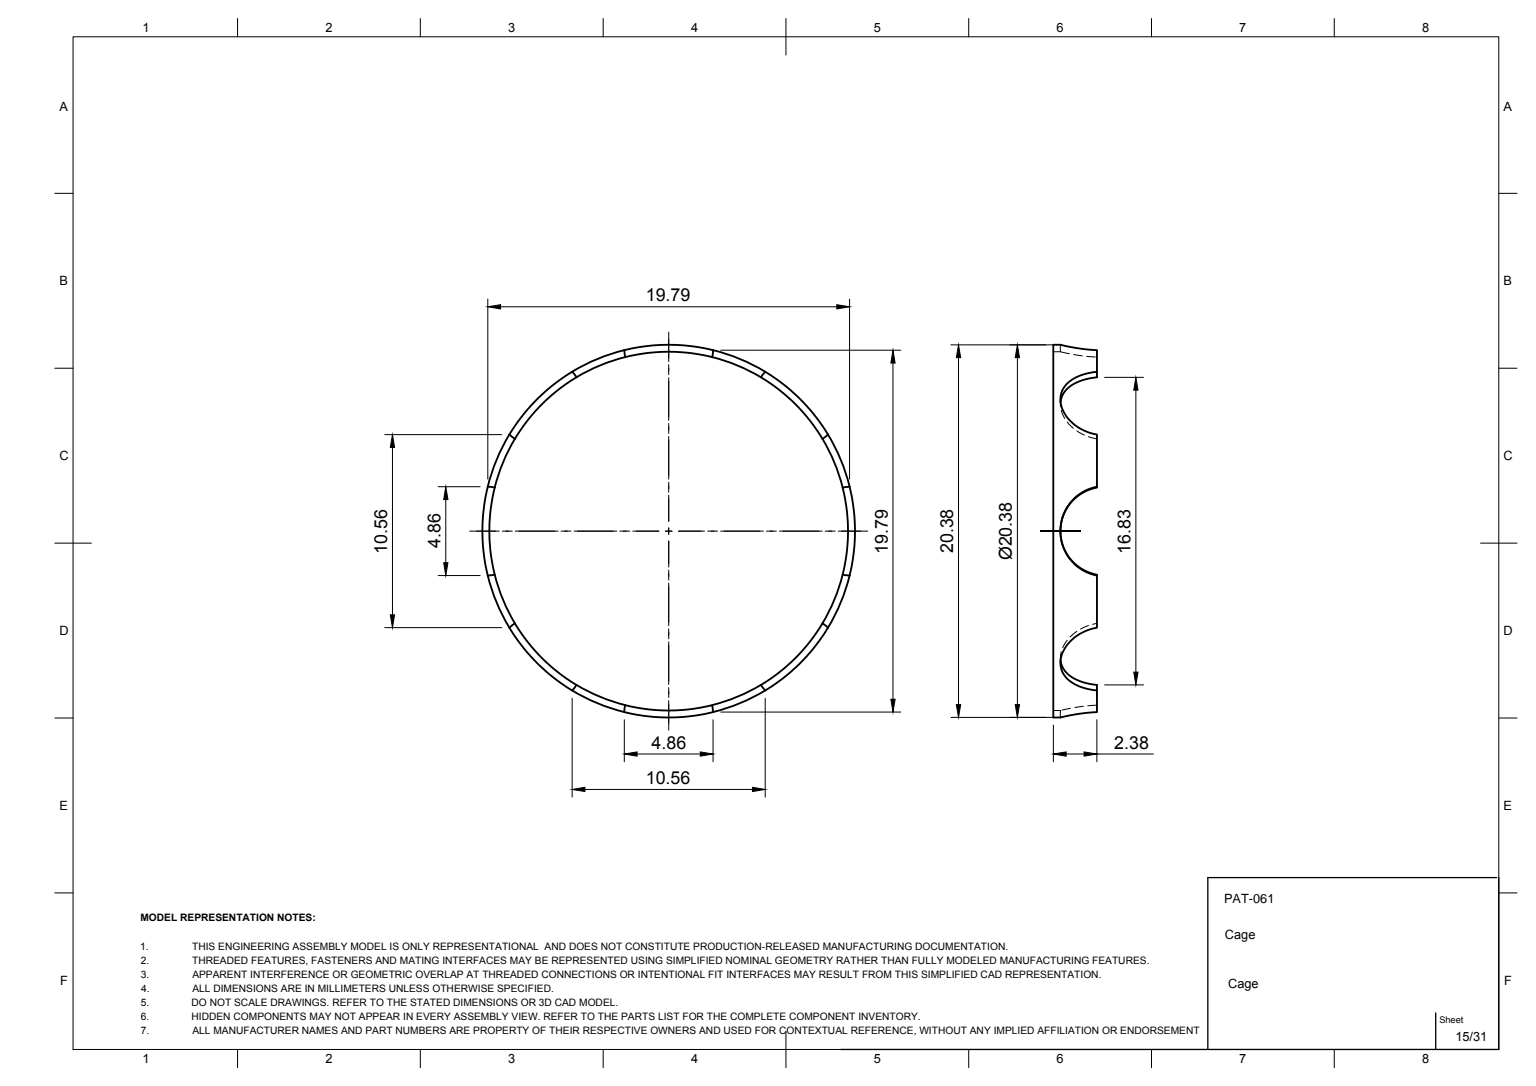
ISO-10303-21;
HEADER;
/* Generated by software containing ST-Developer
 * from STEP Tools, Inc. (www.steptools.com) 
 */

FILE_DESCRIPTION(
/* description */ ('Compact intermittent indexer'),
/* implementation_level */ '2;1');

FILE_NAME(
/* name */ 'Cage.step',
/* time_stamp */ '2026-10-29T16:32:17-07:00',
/* author */ (''),
/* organization */ (''),
/* preprocessor_version */ 'ST-DEVELOPER v20.2',
/* originating_system */ 'Autodesk Translation Framework v15.17.0.0',
/* authorisation */ '');

FILE_SCHEMA (('AUTOMOTIVE_DESIGN { 1 0 10303 214 3 1 1 }'));
ENDSEC;

DATA;
#10=MECHANICAL_DESIGN_GEOMETRIC_PRESENTATION_REPRESENTATION('',(#273),#10837);
#183=SPHERICAL_SURFACE('',#6247,0.247676);
#184=SPHERICAL_SURFACE('',#6263,0.247676);
#185=SPHERICAL_SURFACE('',#6268,0.247676);
#186=SPHERICAL_SURFACE('',#6273,0.247676);
#187=SPHERICAL_SURFACE('',#6278,0.247676);
#188=SPHERICAL_SURFACE('',#6283,0.247676);
#189=SPHERICAL_SURFACE('',#6288,0.247676);
#190=SPHERICAL_SURFACE('',#6296,0.247676);
#218=SHAPE_REPRESENTATION_RELATIONSHIP('SRR','None',#10953,#242);
#242=ADVANCED_BREP_SHAPE_REPRESENTATION('',(#304),#10820);
#273=STYLED_ITEM('',(#11166),#304);
#304=MANIFOLD_SOLID_BREP('Continuous crown cage',#5646);
#321=B_SPLINE_CURVE_WITH_KNOTS('',3,(#9240,#9241,#9242,#9243,#9244,#9245,
#9246,#9247,#9248,#9249,#9250,#9251,#9252,#9253,#9254,#9255,#9256,#9257,
#9258,#9259,#9260,#9261),.UNSPECIFIED.,.F.,.F.,(4,2,2,2,2,2,2,2,2,2,4),
(0.0473477652366656,0.126350602536658,0.189525903804987,0.252701205073317,
0.313298422430275,0.373895639787233,0.434492857144191,0.495090074501149,
0.558265375769478,0.621440677037807,0.7004435143378),.UNSPECIFIED.);
#322=B_SPLINE_CURVE_WITH_KNOTS('',3,(#9265,#9266,#9267,#9268,#9269,#9270,
#9271,#9272,#9273,#9274,#9275,#9276,#9277,#9278,#9279,#9280,#9281,#9282,
#9283,#9284,#9285,#9286),.UNSPECIFIED.,.F.,.F.,(4,2,2,2,2,2,2,2,2,2,4),
(0.0464897534940957,0.0852567806515119,0.170513561303024,0.246687263103517,
0.308657850341199,0.370628437578881,0.432599024816563,0.494569612054245,
0.570743313854739,0.656000094506251,0.694767121663666),.UNSPECIFIED.);
#323=B_SPLINE_CURVE_WITH_KNOTS('',3,(#9292,#9293,#9294,#9295,#9296,#9297,
#9298,#9299,#9300,#9301,#9302,#9303,#9304,#9305,#9306,#9307,#9308,#9309,
#9310,#9311,#9312,#9313),.UNSPECIFIED.,.F.,.F.,(4,2,2,2,2,2,2,2,2,2,4),
(0.0464897534940957,0.0852567806515118,0.170513561303024,0.246687263103517,
0.308657850341199,0.370628437578881,0.432599024816563,0.494569612054245,
0.570743313854738,0.65600009450625,0.694767121663666),.UNSPECIFIED.);
#324=B_SPLINE_CURVE_WITH_KNOTS('',3,(#9317,#9318,#9319,#9320,#9321,#9322,
#9323,#9324,#9325,#9326,#9327,#9328,#9329,#9330,#9331,#9332,#9333,#9334,
#9335,#9336,#9337,#9338),.UNSPECIFIED.,.F.,.F.,(4,2,2,2,2,2,2,2,2,2,4),
(0.0464897534940957,0.0852567806515119,0.170513561303024,0.246687263103517,
0.308657850341199,0.370628437578881,0.432599024816563,0.494569612054245,
0.570743313854739,0.656000094506251,0.694767121663666),.UNSPECIFIED.);
#325=B_SPLINE_CURVE_WITH_KNOTS('',3,(#9342,#9343,#9344,#9345,#9346,#9347,
#9348,#9349,#9350,#9351,#9352,#9353),.UNSPECIFIED.,.F.,.F.,(4,2,2,2,2,4),
(0.0464897534940957,0.0852567806515119,0.170513561303024,0.246687263103517,
0.308657850341199,0.370628437578881),.UNSPECIFIED.);
#326=B_SPLINE_CURVE_WITH_KNOTS('',3,(#9358,#9359,#9360,#9361,#9362,#9363,
#9364,#9365,#9366,#9367,#9368,#9369),.UNSPECIFIED.,.F.,.F.,(4,2,2,2,2,4),
(0.370628437578881,0.432599024816563,0.494569612054245,0.570743313854738,
0.65600009450625,0.694767121663666),.UNSPECIFIED.);
#327=B_SPLINE_CURVE_WITH_KNOTS('',3,(#9373,#9374,#9375,#9376,#9377,#9378,
#9379,#9380,#9381,#9382,#9383,#9384,#9385,#9386,#9387,#9388,#9389,#9390,
#9391,#9392,#9393,#9394),.UNSPECIFIED.,.F.,.F.,(4,2,2,2,2,2,2,2,2,2,4),
(0.0464897534940957,0.0852567806515121,0.170513561303024,0.246687263103518,
0.308657850341199,0.370628437578881,0.432599024816563,0.494569612054245,
0.570743313854738,0.65600009450625,0.694767121663666),.UNSPECIFIED.);
#328=B_SPLINE_CURVE_WITH_KNOTS('',3,(#9398,#9399,#9400,#9401,#9402,#9403,
#9404,#9405,#9406,#9407,#9408,#9409,#9410,#9411,#9412,#9413,#9414,#9415,
#9416,#9417,#9418,#9419),.UNSPECIFIED.,.F.,.F.,(4,2,2,2,2,2,2,2,2,2,4),
(0.0464897534940957,0.0852567806515119,0.170513561303024,0.246687263103517,
0.308657850341199,0.370628437578881,0.432599024816563,0.494569612054245,
0.570743313854738,0.65600009450625,0.694767121663667),.UNSPECIFIED.);
#329=B_SPLINE_CURVE_WITH_KNOTS('',3,(#9423,#9424,#9425,#9426,#9427,#9428,
#9429,#9430,#9431,#9432,#9433,#9434,#9435,#9436,#9437,#9438,#9439,#9440,
#9441,#9442,#9443,#9444),.UNSPECIFIED.,.F.,.F.,(4,2,2,2,2,2,2,2,2,2,4),
(0.0464897534940957,0.0852567806515119,0.170513561303024,0.246687263103517,
0.308657850341199,0.370628437578881,0.432599024816563,0.494569612054245,
0.570743313854738,0.65600009450625,0.694767121663666),.UNSPECIFIED.);
#330=B_SPLINE_CURVE_WITH_KNOTS('',3,(#9448,#9449,#9450,#9451,#9452,#9453,
#9454,#9455,#9456,#9457,#9458,#9459,#9460,#9461,#9462,#9463,#9464,#9465,
#9466,#9467,#9468,#9469),.UNSPECIFIED.,.F.,.F.,(4,2,2,2,2,2,2,2,2,2,4),
(0.0464897534940957,0.0852567806515119,0.170513561303024,0.246687263103517,
0.308657850341199,0.370628437578881,0.432599024816563,0.494569612054245,
0.570743313854739,0.656000094506251,0.694767121663667),.UNSPECIFIED.);
#331=B_SPLINE_CURVE_WITH_KNOTS('',3,(#9477,#9478,#9479,#9480,#9481,#9482,
#9483,#9484,#9485,#9486,#9487,#9488,#9489,#9490,#9491,#9492,#9493,#9494,
#9495,#9496,#9497,#9498),.UNSPECIFIED.,.F.,.F.,(4,2,2,2,2,2,2,2,2,2,4),
(0.0473477652366656,0.126350602536658,0.189525903804987,0.252701205073316,
0.313298422430274,0.373895639787232,0.434492857144191,0.495090074501149,
0.558265375769478,0.621440677037807,0.7004435143378),.UNSPECIFIED.);
#332=B_SPLINE_CURVE_WITH_KNOTS('',3,(#9506,#9507,#9508,#9509,#9510,#9511,
#9512,#9513,#9514,#9515,#9516,#9517,#9518,#9519,#9520,#9521,#9522,#9523,
#9524,#9525,#9526,#9527),.UNSPECIFIED.,.F.,.F.,(4,2,2,2,2,2,2,2,2,2,4),
(0.0473477652366656,0.126350602536658,0.189525903804987,0.252701205073317,
0.313298422430275,0.373895639787233,0.434492857144191,0.495090074501149,
0.558265375769478,0.621440677037807,0.7004435143378),.UNSPECIFIED.);
#333=B_SPLINE_CURVE_WITH_KNOTS('',3,(#9536,#9537,#9538,#9539,#9540,#9541,
#9542,#9543,#9544,#9545,#9546,#9547),.UNSPECIFIED.,.F.,.F.,(4,2,2,2,2,4),
(0.0473477652366656,0.126350602536658,0.189525903804987,0.252701205073316,
0.313298422430275,0.373895639787233),.UNSPECIFIED.);
#334=B_SPLINE_CURVE_WITH_KNOTS('',3,(#9549,#9550,#9551,#9552,#9553,#9554,
#9555,#9556,#9557,#9558,#9559,#9560),.UNSPECIFIED.,.F.,.F.,(4,2,2,2,2,4),
(0.373895639787233,0.434492857144191,0.495090074501149,0.558265375769478,
0.621440677037807,0.7004435143378),.UNSPECIFIED.);
#335=B_SPLINE_CURVE_WITH_KNOTS('',3,(#9567,#9568,#9569,#9570,#9571,#9572,
#9573,#9574,#9575,#9576,#9577,#9578,#9579,#9580,#9581,#9582,#9583,#9584,
#9585,#9586,#9587,#9588),.UNSPECIFIED.,.F.,.F.,(4,2,2,2,2,2,2,2,2,2,4),
(0.0473477652366656,0.126350602536658,0.189525903804987,0.252701205073316,
0.313298422430275,0.373895639787233,0.434492857144191,0.495090074501149,
0.558265375769478,0.621440677037807,0.7004435143378),.UNSPECIFIED.);
#336=B_SPLINE_CURVE_WITH_KNOTS('',3,(#9596,#9597,#9598,#9599,#9600,#9601,
#9602,#9603,#9604,#9605,#9606,#9607,#9608,#9609,#9610,#9611,#9612,#9613,
#9614,#9615,#9616,#9617),.UNSPECIFIED.,.F.,.F.,(4,2,2,2,2,2,2,2,2,2,4),
(0.0473477652366656,0.126350602536658,0.189525903804987,0.252701205073317,
0.313298422430275,0.373895639787233,0.434492857144191,0.495090074501149,
0.558265375769478,0.621440677037807,0.7004435143378),.UNSPECIFIED.);
#337=B_SPLINE_CURVE_WITH_KNOTS('',3,(#9625,#9626,#9627,#9628,#9629,#9630,
#9631,#9632,#9633,#9634,#9635,#9636,#9637,#9638,#9639,#9640,#9641,#9642,
#9643,#9644,#9645,#9646),.UNSPECIFIED.,.F.,.F.,(4,2,2,2,2,2,2,2,2,2,4),
(0.0473477652366656,0.126350602536658,0.189525903804987,0.252701205073316,
0.313298422430275,0.373895639787233,0.434492857144191,0.495090074501149,
0.558265375769478,0.621440677037807,0.7004435143378),.UNSPECIFIED.);
#338=B_SPLINE_CURVE_WITH_KNOTS('',3,(#9655,#9656,#9657,#9658,#9659,#9660,
#9661,#9662,#9663,#9664,#9665,#9666,#9667,#9668,#9669,#9670,#9671,#9672,
#9673,#9674,#9675,#9676),.UNSPECIFIED.,.F.,.F.,(4,2,2,2,2,2,2,2,2,2,4),
(0.0473477652366656,0.126350602536658,0.189525903804987,0.252701205073317,
0.313298422430275,0.373895639787233,0.434492857144191,0.495090074501149,
0.558265375769478,0.621440677037807,0.7004435143378),.UNSPECIFIED.);
#427=FACE_BOUND('',#1222,.T.);
#543=PLANE('',#6260);
#544=PLANE('',#6265);
#545=PLANE('',#6270);
#546=PLANE('',#6275);
#547=PLANE('',#6280);
#548=PLANE('',#6285);
#549=PLANE('',#6294);
#550=PLANE('',#6298);
#551=PLANE('',#6299);
#802=FACE_OUTER_BOUND('',#1204,.T.);
#803=FACE_OUTER_BOUND('',#1205,.T.);
#804=FACE_OUTER_BOUND('',#1206,.T.);
#805=FACE_OUTER_BOUND('',#1207,.T.);
#806=FACE_OUTER_BOUND('',#1208,.T.);
#807=FACE_OUTER_BOUND('',#1209,.T.);
#808=FACE_OUTER_BOUND('',#1210,.T.);
#809=FACE_OUTER_BOUND('',#1211,.T.);
#810=FACE_OUTER_BOUND('',#1212,.T.);
#811=FACE_OUTER_BOUND('',#1213,.T.);
#812=FACE_OUTER_BOUND('',#1214,.T.);
#813=FACE_OUTER_BOUND('',#1215,.T.);
#814=FACE_OUTER_BOUND('',#1216,.T.);
#815=FACE_OUTER_BOUND('',#1217,.T.);
#816=FACE_OUTER_BOUND('',#1218,.T.);
#817=FACE_OUTER_BOUND('',#1219,.T.);
#818=FACE_OUTER_BOUND('',#1220,.T.);
#819=FACE_OUTER_BOUND('',#1221,.T.);
#820=FACE_OUTER_BOUND('',#1223,.T.);
#1204=EDGE_LOOP('',(#4308,#4309,#4310,#4311));
#1205=EDGE_LOOP('',(#4312,#4313,#4314,#4315,#4316,#4317,#4318,#4319,#4320,
#4321,#4322,#4323,#4324,#4325,#4326,#4327,#4328,#4329,#4330,#4331));
#1206=EDGE_LOOP('',(#4332,#4333,#4334,#4335));
#1207=EDGE_LOOP('',(#4336,#4337,#4338,#4339));
#1208=EDGE_LOOP('',(#4340,#4341,#4342,#4343));
#1209=EDGE_LOOP('',(#4344,#4345,#4346,#4347));
#1210=EDGE_LOOP('',(#4348,#4349,#4350,#4351));
#1211=EDGE_LOOP('',(#4352,#4353,#4354,#4355,#4356,#4357));
#1212=EDGE_LOOP('',(#4358,#4359,#4360,#4361));
#1213=EDGE_LOOP('',(#4362,#4363,#4364,#4365));
#1214=EDGE_LOOP('',(#4366,#4367,#4368,#4369));
#1215=EDGE_LOOP('',(#4370,#4371,#4372,#4373));
#1216=EDGE_LOOP('',(#4374,#4375,#4376,#4377));
#1217=EDGE_LOOP('',(#4378,#4379,#4380,#4381));
#1218=EDGE_LOOP('',(#4382,#4383,#4384,#4385,#4386,#4387,#4388,#4389,#4390,
#4391,#4392,#4393,#4394,#4395,#4396,#4397,#4398,#4399,#4400,#4401));
#1219=EDGE_LOOP('',(#4402,#4403,#4404,#4405));
#1220=EDGE_LOOP('',(#4406,#4407,#4408,#4409));
#1221=EDGE_LOOP('',(#4410));
#1222=EDGE_LOOP('',(#4411));
#1223=EDGE_LOOP('',(#4412,#4413,#4414,#4415));
#1574=LINE('',#9355,#1932);
#1575=LINE('',#9651,#1933);
#1932=VECTOR('',#7460,1.019052);
#1933=VECTOR('',#7537,0.980948);
#2304=CIRCLE('',#6248,0.243053047864041);
#2305=CIRCLE('',#6249,0.243053047864041);
#2306=CIRCLE('',#6251,1.019052);
#2307=CIRCLE('',#6252,1.019052);
#2308=CIRCLE('',#6253,1.019052);
#2309=CIRCLE('',#6254,1.019052);
#2310=CIRCLE('',#6255,1.019052);
#2311=CIRCLE('',#6256,1.019052);
#2312=CIRCLE('',#6257,1.019052);
#2313=CIRCLE('',#6258,1.019052);
#2314=CIRCLE('',#6259,1.019052);
#2315=CIRCLE('',#6261,0.980948);
#2316=CIRCLE('',#6262,0.243053047864041);
#2317=CIRCLE('',#6264,0.243053047864041);
#2318=CIRCLE('',#6266,0.980948);
#2319=CIRCLE('',#6267,0.243053047864041);
#2320=CIRCLE('',#6269,0.243053047864041);
#2321=CIRCLE('',#6271,0.980948);
#2322=CIRCLE('',#6272,0.243053047864041);
#2323=CIRCLE('',#6274,0.243053047864041);
#2324=CIRCLE('',#6276,0.980948);
#2325=CIRCLE('',#6277,0.243053047864041);
#2326=CIRCLE('',#6279,0.243053047864041);
#2327=CIRCLE('',#6281,0.980948);
#2328=CIRCLE('',#6282,0.243053047864041);
#2329=CIRCLE('',#6284,0.243053047864041);
#2330=CIRCLE('',#6286,0.980948);
#2331=CIRCLE('',#6287,0.243053047864041);
#2332=CIRCLE('',#6289,0.243053047864041);
#2333=CIRCLE('',#6291,0.980948);
#2334=CIRCLE('',#6292,0.980948);
#2335=CIRCLE('',#6293,0.980948);
#2336=CIRCLE('',#6295,0.243053047864041);
#2337=CIRCLE('',#6297,0.243053047864041);
#2690=VERTEX_POINT('',#9238);
#2691=VERTEX_POINT('',#9239);
#2692=VERTEX_POINT('',#9262);
#2693=VERTEX_POINT('',#9264);
#2694=VERTEX_POINT('',#9289);
#2695=VERTEX_POINT('',#9291);
#2696=VERTEX_POINT('',#9314);
#2697=VERTEX_POINT('',#9316);
#2698=VERTEX_POINT('',#9339);
#2699=VERTEX_POINT('',#9341);
#2700=VERTEX_POINT('',#9354);
#2701=VERTEX_POINT('',#9357);
#2702=VERTEX_POINT('',#9370);
#2703=VERTEX_POINT('',#9372);
#2704=VERTEX_POINT('',#9395);
#2705=VERTEX_POINT('',#9397);
#2706=VERTEX_POINT('',#9420);
#2707=VERTEX_POINT('',#9422);
#2708=VERTEX_POINT('',#9445);
#2709=VERTEX_POINT('',#9447);
#2710=VERTEX_POINT('',#9472);
#2711=VERTEX_POINT('',#9476);
#2712=VERTEX_POINT('',#9501);
#2713=VERTEX_POINT('',#9505);
#2714=VERTEX_POINT('',#9530);
#2715=VERTEX_POINT('',#9534);
#2716=VERTEX_POINT('',#9535);
#2717=VERTEX_POINT('',#9562);
#2718=VERTEX_POINT('',#9566);
#2719=VERTEX_POINT('',#9591);
#2720=VERTEX_POINT('',#9595);
#2721=VERTEX_POINT('',#9620);
#2722=VERTEX_POINT('',#9624);
#2723=VERTEX_POINT('',#9649);
#2724=VERTEX_POINT('',#9652);
#2725=VERTEX_POINT('',#9654);
#3276=EDGE_CURVE('',#2690,#2691,#321,.T.);
#3277=EDGE_CURVE('',#2692,#2690,#2304,.T.);
#3278=EDGE_CURVE('',#2693,#2692,#322,.T.);
#3279=EDGE_CURVE('',#2691,#2693,#2305,.T.);
#3280=EDGE_CURVE('',#2694,#2692,#2306,.T.);
#3281=EDGE_CURVE('',#2694,#2695,#323,.T.);
#3282=EDGE_CURVE('',#2696,#2695,#2307,.T.);
#3283=EDGE_CURVE('',#2696,#2697,#324,.T.);
#3284=EDGE_CURVE('',#2698,#2697,#2308,.T.);
#3285=EDGE_CURVE('',#2698,#2699,#325,.T.);
#3286=EDGE_CURVE('',#2699,#2700,#1574,.T.);
#3287=EDGE_CURVE('',#2700,#2700,#2309,.T.);
#3288=EDGE_CURVE('',#2699,#2701,#326,.T.);
#3289=EDGE_CURVE('',#2702,#2701,#2310,.T.);
#3290=EDGE_CURVE('',#2702,#2703,#327,.T.);
#3291=EDGE_CURVE('',#2704,#2703,#2311,.T.);
#3292=EDGE_CURVE('',#2704,#2705,#328,.T.);
#3293=EDGE_CURVE('',#2706,#2705,#2312,.T.);
#3294=EDGE_CURVE('',#2706,#2707,#329,.T.);
#3295=EDGE_CURVE('',#2708,#2707,#2313,.T.);
#3296=EDGE_CURVE('',#2708,#2709,#330,.T.);
#3297=EDGE_CURVE('',#2693,#2709,#2314,.T.);
#3298=EDGE_CURVE('',#2690,#2710,#2315,.T.);
#3299=EDGE_CURVE('',#2710,#2694,#2316,.T.);
#3300=EDGE_CURVE('',#2711,#2710,#331,.T.);
#3301=EDGE_CURVE('',#2695,#2711,#2317,.T.);
#3302=EDGE_CURVE('',#2711,#2712,#2318,.T.);
#3303=EDGE_CURVE('',#2712,#2696,#2319,.T.);
#3304=EDGE_CURVE('',#2713,#2712,#332,.T.);
#3305=EDGE_CURVE('',#2697,#2713,#2320,.T.);
#3306=EDGE_CURVE('',#2713,#2714,#2321,.T.);
#3307=EDGE_CURVE('',#2714,#2698,#2322,.T.);
#3308=EDGE_CURVE('',#2715,#2716,#333,.T.);
#3309=EDGE_CURVE('',#2701,#2715,#2323,.T.);
#3310=EDGE_CURVE('',#2716,#2714,#334,.T.);
#3311=EDGE_CURVE('',#2715,#2717,#2324,.T.);
#3312=EDGE_CURVE('',#2717,#2702,#2325,.T.);
#3313=EDGE_CURVE('',#2718,#2717,#335,.T.);
#3314=EDGE_CURVE('',#2703,#2718,#2326,.T.);
#3315=EDGE_CURVE('',#2718,#2719,#2327,.T.);
#3316=EDGE_CURVE('',#2719,#2704,#2328,.T.);
#3317=EDGE_CURVE('',#2720,#2719,#336,.T.);
#3318=EDGE_CURVE('',#2705,#2720,#2329,.T.);
#3319=EDGE_CURVE('',#2720,#2721,#2330,.T.);
#3320=EDGE_CURVE('',#2721,#2706,#2331,.T.);
#3321=EDGE_CURVE('',#2722,#2721,#337,.T.);
#3322=EDGE_CURVE('',#2707,#2722,#2332,.T.);
#3323=EDGE_CURVE('',#2723,#2723,#2333,.T.);
#3324=EDGE_CURVE('',#2723,#2716,#1575,.T.);
#3325=EDGE_CURVE('',#2724,#2691,#2334,.T.);
#3326=EDGE_CURVE('',#2724,#2725,#338,.T.);
#3327=EDGE_CURVE('',#2722,#2725,#2335,.T.);
#3328=EDGE_CURVE('',#2709,#2724,#2336,.T.);
#3329=EDGE_CURVE('',#2725,#2708,#2337,.T.);
#4308=ORIENTED_EDGE('',*,*,#3276,.F.);
#4309=ORIENTED_EDGE('',*,*,#3277,.F.);
#4310=ORIENTED_EDGE('',*,*,#3278,.F.);
#4311=ORIENTED_EDGE('',*,*,#3279,.F.);
#4312=ORIENTED_EDGE('',*,*,#3278,.T.);
#4313=ORIENTED_EDGE('',*,*,#3280,.F.);
#4314=ORIENTED_EDGE('',*,*,#3281,.T.);
#4315=ORIENTED_EDGE('',*,*,#3282,.F.);
#4316=ORIENTED_EDGE('',*,*,#3283,.T.);
#4317=ORIENTED_EDGE('',*,*,#3284,.F.);
#4318=ORIENTED_EDGE('',*,*,#3285,.T.);
#4319=ORIENTED_EDGE('',*,*,#3286,.T.);
#4320=ORIENTED_EDGE('',*,*,#3287,.F.);
#4321=ORIENTED_EDGE('',*,*,#3286,.F.);
#4322=ORIENTED_EDGE('',*,*,#3288,.T.);
#4323=ORIENTED_EDGE('',*,*,#3289,.F.);
#4324=ORIENTED_EDGE('',*,*,#3290,.T.);
#4325=ORIENTED_EDGE('',*,*,#3291,.F.);
#4326=ORIENTED_EDGE('',*,*,#3292,.T.);
#4327=ORIENTED_EDGE('',*,*,#3293,.F.);
#4328=ORIENTED_EDGE('',*,*,#3294,.T.);
#4329=ORIENTED_EDGE('',*,*,#3295,.F.);
#4330=ORIENTED_EDGE('',*,*,#3296,.T.);
#4331=ORIENTED_EDGE('',*,*,#3297,.F.);
#4332=ORIENTED_EDGE('',*,*,#3277,.T.);
#4333=ORIENTED_EDGE('',*,*,#3298,.T.);
#4334=ORIENTED_EDGE('',*,*,#3299,.T.);
#4335=ORIENTED_EDGE('',*,*,#3280,.T.);
#4336=ORIENTED_EDGE('',*,*,#3300,.F.);
#4337=ORIENTED_EDGE('',*,*,#3301,.F.);
#4338=ORIENTED_EDGE('',*,*,#3281,.F.);
#4339=ORIENTED_EDGE('',*,*,#3299,.F.);
#4340=ORIENTED_EDGE('',*,*,#3301,.T.);
#4341=ORIENTED_EDGE('',*,*,#3302,.T.);
#4342=ORIENTED_EDGE('',*,*,#3303,.T.);
#4343=ORIENTED_EDGE('',*,*,#3282,.T.);
#4344=ORIENTED_EDGE('',*,*,#3304,.F.);
#4345=ORIENTED_EDGE('',*,*,#3305,.F.);
#4346=ORIENTED_EDGE('',*,*,#3283,.F.);
#4347=ORIENTED_EDGE('',*,*,#3303,.F.);
#4348=ORIENTED_EDGE('',*,*,#3305,.T.);
#4349=ORIENTED_EDGE('',*,*,#3306,.T.);
#4350=ORIENTED_EDGE('',*,*,#3307,.T.);
#4351=ORIENTED_EDGE('',*,*,#3284,.T.);
#4352=ORIENTED_EDGE('',*,*,#3308,.F.);
#4353=ORIENTED_EDGE('',*,*,#3309,.F.);
#4354=ORIENTED_EDGE('',*,*,#3288,.F.);
#4355=ORIENTED_EDGE('',*,*,#3285,.F.);
#4356=ORIENTED_EDGE('',*,*,#3307,.F.);
#4357=ORIENTED_EDGE('',*,*,#3310,.F.);
#4358=ORIENTED_EDGE('',*,*,#3309,.T.);
#4359=ORIENTED_EDGE('',*,*,#3311,.T.);
#4360=ORIENTED_EDGE('',*,*,#3312,.T.);
#4361=ORIENTED_EDGE('',*,*,#3289,.T.);
#4362=ORIENTED_EDGE('',*,*,#3313,.F.);
#4363=ORIENTED_EDGE('',*,*,#3314,.F.);
#4364=ORIENTED_EDGE('',*,*,#3290,.F.);
#4365=ORIENTED_EDGE('',*,*,#3312,.F.);
#4366=ORIENTED_EDGE('',*,*,#3314,.T.);
#4367=ORIENTED_EDGE('',*,*,#3315,.T.);
#4368=ORIENTED_EDGE('',*,*,#3316,.T.);
#4369=ORIENTED_EDGE('',*,*,#3291,.T.);
#4370=ORIENTED_EDGE('',*,*,#3317,.F.);
#4371=ORIENTED_EDGE('',*,*,#3318,.F.);
#4372=ORIENTED_EDGE('',*,*,#3292,.F.);
#4373=ORIENTED_EDGE('',*,*,#3316,.F.);
#4374=ORIENTED_EDGE('',*,*,#3318,.T.);
#4375=ORIENTED_EDGE('',*,*,#3319,.T.);
#4376=ORIENTED_EDGE('',*,*,#3320,.T.);
#4377=ORIENTED_EDGE('',*,*,#3293,.T.);
#4378=ORIENTED_EDGE('',*,*,#3294,.F.);
#4379=ORIENTED_EDGE('',*,*,#3320,.F.);
#4380=ORIENTED_EDGE('',*,*,#3321,.F.);
#4381=ORIENTED_EDGE('',*,*,#3322,.F.);
#4382=ORIENTED_EDGE('',*,*,#3323,.F.);
#4383=ORIENTED_EDGE('',*,*,#3324,.T.);
#4384=ORIENTED_EDGE('',*,*,#3310,.T.);
#4385=ORIENTED_EDGE('',*,*,#3306,.F.);
#4386=ORIENTED_EDGE('',*,*,#3304,.T.);
#4387=ORIENTED_EDGE('',*,*,#3302,.F.);
#4388=ORIENTED_EDGE('',*,*,#3300,.T.);
#4389=ORIENTED_EDGE('',*,*,#3298,.F.);
#4390=ORIENTED_EDGE('',*,*,#3276,.T.);
#4391=ORIENTED_EDGE('',*,*,#3325,.F.);
#4392=ORIENTED_EDGE('',*,*,#3326,.T.);
#4393=ORIENTED_EDGE('',*,*,#3327,.F.);
#4394=ORIENTED_EDGE('',*,*,#3321,.T.);
#4395=ORIENTED_EDGE('',*,*,#3319,.F.);
#4396=ORIENTED_EDGE('',*,*,#3317,.T.);
#4397=ORIENTED_EDGE('',*,*,#3315,.F.);
#4398=ORIENTED_EDGE('',*,*,#3313,.T.);
#4399=ORIENTED_EDGE('',*,*,#3311,.F.);
#4400=ORIENTED_EDGE('',*,*,#3308,.T.);
#4401=ORIENTED_EDGE('',*,*,#3324,.F.);
#4402=ORIENTED_EDGE('',*,*,#3279,.T.);
#4403=ORIENTED_EDGE('',*,*,#3297,.T.);
#4404=ORIENTED_EDGE('',*,*,#3328,.T.);
#4405=ORIENTED_EDGE('',*,*,#3325,.T.);
#4406=ORIENTED_EDGE('',*,*,#3296,.F.);
#4407=ORIENTED_EDGE('',*,*,#3329,.F.);
#4408=ORIENTED_EDGE('',*,*,#3326,.F.);
#4409=ORIENTED_EDGE('',*,*,#3328,.F.);
#4410=ORIENTED_EDGE('',*,*,#3287,.T.);
#4411=ORIENTED_EDGE('',*,*,#3323,.T.);
#4412=ORIENTED_EDGE('',*,*,#3322,.T.);
#4413=ORIENTED_EDGE('',*,*,#3327,.T.);
#4414=ORIENTED_EDGE('',*,*,#3329,.T.);
#4415=ORIENTED_EDGE('',*,*,#3295,.T.);
#5232=CYLINDRICAL_SURFACE('',#6250,1.019052);
#5233=CYLINDRICAL_SURFACE('',#6290,0.980948);
#5445=ADVANCED_FACE('',(#802),#183,.F.);
#5446=ADVANCED_FACE('',(#803),#5232,.T.);
#5447=ADVANCED_FACE('',(#804),#543,.T.);
#5448=ADVANCED_FACE('',(#805),#184,.F.);
#5449=ADVANCED_FACE('',(#806),#544,.T.);
#5450=ADVANCED_FACE('',(#807),#185,.F.);
#5451=ADVANCED_FACE('',(#808),#545,.T.);
#5452=ADVANCED_FACE('',(#809),#186,.F.);
#5453=ADVANCED_FACE('',(#810),#546,.T.);
#5454=ADVANCED_FACE('',(#811),#187,.F.);
#5455=ADVANCED_FACE('',(#812),#547,.T.);
#5456=ADVANCED_FACE('',(#813),#188,.F.);
#5457=ADVANCED_FACE('',(#814),#548,.T.);
#5458=ADVANCED_FACE('',(#815),#189,.F.);
#5459=ADVANCED_FACE('',(#816),#5233,.F.);
#5460=ADVANCED_FACE('',(#817),#549,.T.);
#5461=ADVANCED_FACE('',(#818),#190,.F.);
#5462=ADVANCED_FACE('',(#819,#427),#550,.T.);
#5463=ADVANCED_FACE('',(#820),#551,.T.);
#5646=CLOSED_SHELL('',(#5445,#5446,#5447,#5448,#5449,#5450,#5451,#5452,
#5453,#5454,#5455,#5456,#5457,#5458,#5459,#5460,#5461,#5462,#5463));
#6246=AXIS2_PLACEMENT_3D('',#9236,#7444,#7445);
#6247=AXIS2_PLACEMENT_3D('',#9237,#7446,#7447);
#6248=AXIS2_PLACEMENT_3D('',#9263,#7448,#7449);
#6249=AXIS2_PLACEMENT_3D('',#9287,#7450,#7451);
#6250=AXIS2_PLACEMENT_3D('',#9288,#7452,#7453);
#6251=AXIS2_PLACEMENT_3D('',#9290,#7454,#7455);
#6252=AXIS2_PLACEMENT_3D('',#9315,#7456,#7457);
#6253=AXIS2_PLACEMENT_3D('',#9340,#7458,#7459);
#6254=AXIS2_PLACEMENT_3D('',#9356,#7461,#7462);
#6255=AXIS2_PLACEMENT_3D('',#9371,#7463,#7464);
#6256=AXIS2_PLACEMENT_3D('',#9396,#7465,#7466);
#6257=AXIS2_PLACEMENT_3D('',#9421,#7467,#7468);
#6258=AXIS2_PLACEMENT_3D('',#9446,#7469,#7470);
#6259=AXIS2_PLACEMENT_3D('',#9470,#7471,#7472);
#6260=AXIS2_PLACEMENT_3D('',#9471,#7473,#7474);
#6261=AXIS2_PLACEMENT_3D('',#9473,#7475,#7476);
#6262=AXIS2_PLACEMENT_3D('',#9474,#7477,#7478);
#6263=AXIS2_PLACEMENT_3D('',#9475,#7479,#7480);
#6264=AXIS2_PLACEMENT_3D('',#9499,#7481,#7482);
#6265=AXIS2_PLACEMENT_3D('',#9500,#7483,#7484);
#6266=AXIS2_PLACEMENT_3D('',#9502,#7485,#7486);
#6267=AXIS2_PLACEMENT_3D('',#9503,#7487,#7488);
#6268=AXIS2_PLACEMENT_3D('',#9504,#7489,#7490);
#6269=AXIS2_PLACEMENT_3D('',#9528,#7491,#7492);
#6270=AXIS2_PLACEMENT_3D('',#9529,#7493,#7494);
#6271=AXIS2_PLACEMENT_3D('',#9531,#7495,#7496);
#6272=AXIS2_PLACEMENT_3D('',#9532,#7497,#7498);
#6273=AXIS2_PLACEMENT_3D('',#9533,#7499,#7500);
#6274=AXIS2_PLACEMENT_3D('',#9548,#7501,#7502);
#6275=AXIS2_PLACEMENT_3D('',#9561,#7503,#7504);
#6276=AXIS2_PLACEMENT_3D('',#9563,#7505,#7506);
#6277=AXIS2_PLACEMENT_3D('',#9564,#7507,#7508);
#6278=AXIS2_PLACEMENT_3D('',#9565,#7509,#7510);
#6279=AXIS2_PLACEMENT_3D('',#9589,#7511,#7512);
#6280=AXIS2_PLACEMENT_3D('',#9590,#7513,#7514);
#6281=AXIS2_PLACEMENT_3D('',#9592,#7515,#7516);
#6282=AXIS2_PLACEMENT_3D('',#9593,#7517,#7518);
#6283=AXIS2_PLACEMENT_3D('',#9594,#7519,#7520);
#6284=AXIS2_PLACEMENT_3D('',#9618,#7521,#7522);
#6285=AXIS2_PLACEMENT_3D('',#9619,#7523,#7524);
#6286=AXIS2_PLACEMENT_3D('',#9621,#7525,#7526);
#6287=AXIS2_PLACEMENT_3D('',#9622,#7527,#7528);
#6288=AXIS2_PLACEMENT_3D('',#9623,#7529,#7530);
#6289=AXIS2_PLACEMENT_3D('',#9647,#7531,#7532);
#6290=AXIS2_PLACEMENT_3D('',#9648,#7533,#7534);
#6291=AXIS2_PLACEMENT_3D('',#9650,#7535,#7536);
#6292=AXIS2_PLACEMENT_3D('',#9653,#7538,#7539);
#6293=AXIS2_PLACEMENT_3D('',#9677,#7540,#7541);
#6294=AXIS2_PLACEMENT_3D('',#9678,#7542,#7543);
#6295=AXIS2_PLACEMENT_3D('',#9679,#7544,#7545);
#6296=AXIS2_PLACEMENT_3D('',#9680,#7546,#7547);
#6297=AXIS2_PLACEMENT_3D('',#9681,#7548,#7549);
#6298=AXIS2_PLACEMENT_3D('',#9682,#7550,#7551);
#6299=AXIS2_PLACEMENT_3D('',#9683,#7552,#7553);
#7444=DIRECTION('axis',(0.,0.,1.));
#7445=DIRECTION('refdir',(1.,0.,0.));
#7446=DIRECTION('center_axis',(0.,0.,1.));
#7447=DIRECTION('ref_axis',(1.,0.,0.));
#7448=DIRECTION('center_axis',(0.,-1.,0.));
#7449=DIRECTION('ref_axis',(0.,0.,-1.));
#7450=DIRECTION('center_axis',(0.,-1.,0.));
#7451=DIRECTION('ref_axis',(0.,0.,-1.));
#7452=DIRECTION('center_axis',(0.,1.,0.));
#7453=DIRECTION('ref_axis',(1.,0.,0.));
#7454=DIRECTION('center_axis',(0.,1.,0.));
#7455=DIRECTION('ref_axis',(1.,0.,0.));
#7456=DIRECTION('center_axis',(0.,1.,0.));
#7457=DIRECTION('ref_axis',(1.,0.,0.));
#7458=DIRECTION('center_axis',(0.,1.,0.));
#7459=DIRECTION('ref_axis',(1.,0.,0.));
#7460=DIRECTION('',(0.,-1.,0.));
#7461=DIRECTION('center_axis',(0.,-1.,0.));
#7462=DIRECTION('ref_axis',(1.,0.,0.));
#7463=DIRECTION('center_axis',(0.,1.,0.));
#7464=DIRECTION('ref_axis',(1.,0.,0.));
#7465=DIRECTION('center_axis',(0.,1.,0.));
#7466=DIRECTION('ref_axis',(1.,0.,0.));
#7467=DIRECTION('center_axis',(0.,1.,0.));
#7468=DIRECTION('ref_axis',(1.,0.,0.));
#7469=DIRECTION('center_axis',(0.,1.,0.));
#7470=DIRECTION('ref_axis',(1.,0.,0.));
#7471=DIRECTION('center_axis',(0.,1.,0.));
#7472=DIRECTION('ref_axis',(1.,0.,0.));
#7473=DIRECTION('center_axis',(0.,1.,0.));
#7474=DIRECTION('ref_axis',(1.,0.,0.));
#7475=DIRECTION('center_axis',(0.,-1.,0.));
#7476=DIRECTION('ref_axis',(1.,0.,0.));
#7477=DIRECTION('center_axis',(0.,-1.,0.));
#7478=DIRECTION('ref_axis',(0.,0.,-1.));
#7479=DIRECTION('center_axis',(6.12323399573677E-17,0.,1.));
#7480=DIRECTION('ref_axis',(1.,0.,0.));
#7481=DIRECTION('center_axis',(0.,-1.,0.));
#7482=DIRECTION('ref_axis',(0.,0.,-1.));
#7483=DIRECTION('center_axis',(0.,1.,0.));
#7484=DIRECTION('ref_axis',(1.,0.,0.));
#7485=DIRECTION('center_axis',(0.,-1.,0.));
#7486=DIRECTION('ref_axis',(1.,0.,0.));
#7487=DIRECTION('center_axis',(0.,-1.,0.));
#7488=DIRECTION('ref_axis',(0.,0.,-1.));
#7489=DIRECTION('center_axis',(0.,0.,1.));
#7490=DIRECTION('ref_axis',(1.,0.,0.));
#7491=DIRECTION('center_axis',(0.,-1.,0.));
#7492=DIRECTION('ref_axis',(0.,0.,-1.));
#7493=DIRECTION('center_axis',(0.,1.,0.));
#7494=DIRECTION('ref_axis',(1.,0.,0.));
#7495=DIRECTION('center_axis',(0.,-1.,0.));
#7496=DIRECTION('ref_axis',(1.,0.,0.));
#7497=DIRECTION('center_axis',(0.,-1.,0.));
#7498=DIRECTION('ref_axis',(0.,0.,-1.));
#7499=DIRECTION('center_axis',(0.,0.,1.));
#7500=DIRECTION('ref_axis',(1.,0.,0.));
#7501=DIRECTION('center_axis',(0.,-1.,0.));
#7502=DIRECTION('ref_axis',(0.,0.,-1.));
#7503=DIRECTION('center_axis',(0.,1.,0.));
#7504=DIRECTION('ref_axis',(1.,0.,0.));
#7505=DIRECTION('center_axis',(0.,-1.,0.));
#7506=DIRECTION('ref_axis',(1.,0.,0.));
#7507=DIRECTION('center_axis',(0.,-1.,0.));
#7508=DIRECTION('ref_axis',(0.,0.,-1.));
#7509=DIRECTION('center_axis',(0.,0.,1.));
#7510=DIRECTION('ref_axis',(1.,0.,0.));
#7511=DIRECTION('center_axis',(0.,-1.,0.));
#7512=DIRECTION('ref_axis',(0.,0.,-1.));
#7513=DIRECTION('center_axis',(0.,1.,0.));
#7514=DIRECTION('ref_axis',(1.,0.,0.));
#7515=DIRECTION('center_axis',(0.,-1.,0.));
#7516=DIRECTION('ref_axis',(1.,0.,0.));
#7517=DIRECTION('center_axis',(0.,-1.,0.));
#7518=DIRECTION('ref_axis',(0.,0.,-1.));
#7519=DIRECTION('center_axis',(6.12323399573676E-17,0.,1.));
#7520=DIRECTION('ref_axis',(1.,0.,0.));
#7521=DIRECTION('center_axis',(0.,-1.,0.));
#7522=DIRECTION('ref_axis',(0.,0.,-1.));
#7523=DIRECTION('center_axis',(0.,1.,0.));
#7524=DIRECTION('ref_axis',(1.,0.,0.));
#7525=DIRECTION('center_axis',(0.,-1.,0.));
#7526=DIRECTION('ref_axis',(1.,0.,0.));
#7527=DIRECTION('center_axis',(0.,-1.,0.));
#7528=DIRECTION('ref_axis',(0.,0.,-1.));
#7529=DIRECTION('center_axis',(0.,0.,1.));
#7530=DIRECTION('ref_axis',(1.,0.,0.));
#7531=DIRECTION('center_axis',(0.,-1.,0.));
#7532=DIRECTION('ref_axis',(0.,0.,-1.));
#7533=DIRECTION('center_axis',(0.,1.,0.));
#7534=DIRECTION('ref_axis',(1.,0.,0.));
#7535=DIRECTION('center_axis',(0.,1.,0.));
#7536=DIRECTION('ref_axis',(1.,0.,0.));
#7537=DIRECTION('',(0.,1.,0.));
#7538=DIRECTION('center_axis',(0.,-1.,0.));
#7539=DIRECTION('ref_axis',(1.,0.,0.));
#7540=DIRECTION('center_axis',(0.,-1.,0.));
#7541=DIRECTION('ref_axis',(1.,0.,0.));
#7542=DIRECTION('center_axis',(0.,1.,0.));
#7543=DIRECTION('ref_axis',(1.,0.,0.));
#7544=DIRECTION('center_axis',(0.,-1.,0.));
#7545=DIRECTION('ref_axis',(0.,0.,-1.));
#7546=DIRECTION('center_axis',(0.,0.,1.));
#7547=DIRECTION('ref_axis',(1.,0.,0.));
#7548=DIRECTION('center_axis',(0.,-1.,0.));
#7549=DIRECTION('ref_axis',(0.,0.,-1.));
#7550=DIRECTION('center_axis',(0.,-1.,0.));
#7551=DIRECTION('ref_axis',(-1.,0.,0.));
#7552=DIRECTION('center_axis',(0.,1.,0.));
#7553=DIRECTION('ref_axis',(1.,0.,0.));
#9236=CARTESIAN_POINT('',(0.,0.,0.));
#9237=CARTESIAN_POINT('Origin',(0.707106781186547,0.,0.707106781186548));
#9238=CARTESIAN_POINT('',(0.504455939115715,-0.04763,0.841298510752802));
#9239=CARTESIAN_POINT('',(0.841298510752802,-0.04763,0.504455939115715));
#9240=CARTESIAN_POINT('Ctrl Pts',(0.504455939115715,-0.04763,0.841298510752802));
#9241=CARTESIAN_POINT('Ctrl Pts',(0.508899795931835,-0.0740444353928835,
0.838633903678357));
#9242=CARTESIAN_POINT('Ctrl Pts',(0.517157748491652,-0.0999305678883309,
0.833661031856294));
#9243=CARTESIAN_POINT('Ctrl Pts',(0.537715343527944,-0.142345102874864,
0.820511285096538));
#9244=CARTESIAN_POINT('Ctrl Pts',(0.548874290046456,-0.159766064500479,
0.813159949759));
#9245=CARTESIAN_POINT('Ctrl Pts',(0.573915184558107,-0.190326085855194,
0.795684265985089));
#9246=CARTESIAN_POINT('Ctrl Pts',(0.587792702767295,-0.203463743702801,
0.78555112003688));
#9247=CARTESIAN_POINT('Ctrl Pts',(0.615966552324775,-0.224161999508995,
0.763642258217233));
#9248=CARTESIAN_POINT('Ctrl Pts',(0.631684198665438,-0.232861760990032,
0.750785745543687));
#9249=CARTESIAN_POINT('Ctrl Pts',(0.663382628119203,-0.244251601209411,
0.722929908501543));
#9250=CARTESIAN_POINT('Ctrl Pts',(0.679352081686668,-0.246942143572133,
0.707917883896095));
#9251=CARTESIAN_POINT('Ctrl Pts',(0.707917883896095,-0.246942143572133,
0.679352081686668));
#9252=CARTESIAN_POINT('Ctrl Pts',(0.722929908501543,-0.244251601209411,
0.663382628119203));
#9253=CARTESIAN_POINT('Ctrl Pts',(0.750785745543687,-0.232861760990032,
0.631684198665439));
#9254=CARTESIAN_POINT('Ctrl Pts',(0.763642258217232,-0.224161999508995,
0.615966552324775));
#9255=CARTESIAN_POINT('Ctrl Pts',(0.78555112003688,-0.203463743702801,0.587792702767295));
#9256=CARTESIAN_POINT('Ctrl Pts',(0.795684265985088,-0.190326085855194,
0.573915184558108));
#9257=CARTESIAN_POINT('Ctrl Pts',(0.813159949759,-0.15976606450048,0.548874290046456));
#9258=CARTESIAN_POINT('Ctrl Pts',(0.820511285096538,-0.142345102874864,
0.537715343527944));
#9259=CARTESIAN_POINT('Ctrl Pts',(0.833661031856294,-0.099930567888331,
0.517157748491653));
#9260=CARTESIAN_POINT('Ctrl Pts',(0.838633903678357,-0.0740444353928835,
0.508899795931835));
#9261=CARTESIAN_POINT('Ctrl Pts',(0.841298510752801,-0.0476299999999999,
0.504455939115715));
#9262=CARTESIAN_POINT('',(0.528110872004958,-0.04763,0.871530771444223));
#9263=CARTESIAN_POINT('Origin',(0.707106781186547,-0.04763,0.707106781186548));
#9264=CARTESIAN_POINT('',(0.871530771444223,-0.04763,0.528110872004959));
#9265=CARTESIAN_POINT('Ctrl Pts',(0.871530771444223,-0.0476300000000001,
0.528110872004958));
#9266=CARTESIAN_POINT('Ctrl Pts',(0.87014664509073,-0.0609922781173483,
0.530395067942936));
#9267=CARTESIAN_POINT('Ctrl Pts',(0.868149331745851,-0.0742967091364493,
0.533674141594226));
#9268=CARTESIAN_POINT('Ctrl Pts',(0.85981294420286,-0.115492077056649,0.54708917182331));
#9269=CARTESIAN_POINT('Ctrl Pts',(0.850993704737257,-0.141695629206859,
0.560922177770136));
#9270=CARTESIAN_POINT('Ctrl Pts',(0.830754510485543,-0.181890537957859,
0.590422647829571));
#9271=CARTESIAN_POINT('Ctrl Pts',(0.816896541396381,-0.201072148666545,
0.609616703125488));
#9272=CARTESIAN_POINT('Ctrl Pts',(0.792310597819928,-0.223955109275652,
0.641117951819998));
#9273=CARTESIAN_POINT('Ctrl Pts',(0.779109323683612,-0.232742381310829,
0.657208095763053));
#9274=CARTESIAN_POINT('Ctrl Pts',(0.750552691816206,-0.244234834628584,
0.68964083160521));
#9275=CARTESIAN_POINT('Ctrl Pts',(0.735185187071673,-0.246942143572133,
0.705971972091755));
#9276=CARTESIAN_POINT('Ctrl Pts',(0.705971972091754,-0.246942143572133,
0.735185187071673));
#9277=CARTESIAN_POINT('Ctrl Pts',(0.689640831605209,-0.244234834628584,
0.750552691816206));
#9278=CARTESIAN_POINT('Ctrl Pts',(0.657208095763052,-0.232742381310829,
0.779109323683612));
#9279=CARTESIAN_POINT('Ctrl Pts',(0.641117951819998,-0.223955109275652,
0.792310597819928));
#9280=CARTESIAN_POINT('Ctrl Pts',(0.609616703125487,-0.201072148666545,
0.816896541396382));
#9281=CARTESIAN_POINT('Ctrl Pts',(0.590422647829571,-0.181890537957858,
0.830754510485544));
#9282=CARTESIAN_POINT('Ctrl Pts',(0.560922177770135,-0.141695629206858,
0.850993704737257));
#9283=CARTESIAN_POINT('Ctrl Pts',(0.547089171823309,-0.115492077056649,
0.859812944202861));
#9284=CARTESIAN_POINT('Ctrl Pts',(0.533674141594226,-0.0742967091364491,
0.868149331745852));
#9285=CARTESIAN_POINT('Ctrl Pts',(0.530395067942936,-0.0609922781173483,
0.870146645090731));
#9286=CARTESIAN_POINT('Ctrl Pts',(0.528110872004958,-0.0476300000000001,
0.871530771444223));
#9287=CARTESIAN_POINT('Origin',(0.707106781186547,-0.04763,0.707106781186548));
#9288=CARTESIAN_POINT('Origin',(0.,-0.166705,0.));
#9289=CARTESIAN_POINT('',(0.242834539687906,-0.04763,0.989696097314));
#9290=CARTESIAN_POINT('Origin',(0.,-0.04763,0.));
#9291=CARTESIAN_POINT('',(-0.242834539687907,-0.04763,0.989696097314));
#9292=CARTESIAN_POINT('Ctrl Pts',(0.242834539687906,-0.04763,0.989696097314));
#9293=CARTESIAN_POINT('Ctrl Pts',(0.24024064412003,-0.0609922781173483,
0.990332542620729));
#9294=CARTESIAN_POINT('Ctrl Pts',(0.236509675094874,-0.0742967091364492,
0.991238884025248));
#9295=CARTESIAN_POINT('Ctrl Pts',(0.221129100087819,-0.115492077056649,
0.994830026707808));
#9296=CARTESIAN_POINT('Ctrl Pts',(0.205111543747588,-0.141695629206859,
0.998375294985966));
#9297=CARTESIAN_POINT('Ctrl Pts',(0.169940289819232,-0.181890537957859,
1.00492400591205));
#9298=CARTESIAN_POINT('Ctrl Pts',(0.1465689792446,-0.201072148666545,1.00869718865384));
#9299=CARTESIAN_POINT('Ctrl Pts',(0.106909345252087,-0.223955109275652,
1.01358704779679));
#9300=CARTESIAN_POINT('Ctrl Pts',(0.0861971848975941,-0.232742381310829,
1.0156297872271));
#9301=CARTESIAN_POINT('Ctrl Pts',(0.0430711894098822,-0.244234834628584,
1.01837060663223));
#9302=CARTESIAN_POINT('Ctrl Pts',(0.0206568624125605,-0.246942143572133,
1.019052));
#9303=CARTESIAN_POINT('Ctrl Pts',(-0.0206568624125608,-0.246942143572133,
1.019052));
#9304=CARTESIAN_POINT('Ctrl Pts',(-0.0430711894098825,-0.244234834628584,
1.01837060663223));
#9305=CARTESIAN_POINT('Ctrl Pts',(-0.0861971848975943,-0.232742381310829,
1.0156297872271));
#9306=CARTESIAN_POINT('Ctrl Pts',(-0.106909345252088,-0.223955109275652,
1.01358704779679));
#9307=CARTESIAN_POINT('Ctrl Pts',(-0.1465689792446,-0.201072148666545,1.00869718865384));
#9308=CARTESIAN_POINT('Ctrl Pts',(-0.169940289819232,-0.181890537957859,
1.00492400591205));
#9309=CARTESIAN_POINT('Ctrl Pts',(-0.205111543747588,-0.141695629206859,
0.998375294985966));
#9310=CARTESIAN_POINT('Ctrl Pts',(-0.221129100087819,-0.115492077056649,
0.994830026707808));
#9311=CARTESIAN_POINT('Ctrl Pts',(-0.236509675094875,-0.0742967091364493,
0.991238884025248));
#9312=CARTESIAN_POINT('Ctrl Pts',(-0.24024064412003,-0.0609922781173483,
0.990332542620729));
#9313=CARTESIAN_POINT('Ctrl Pts',(-0.242834539687907,-0.04763,0.989696097314));
#9314=CARTESIAN_POINT('',(-0.528110872004959,-0.04763,0.871530771444223));
#9315=CARTESIAN_POINT('Origin',(0.,-0.04763,0.));
#9316=CARTESIAN_POINT('',(-0.871530771444223,-0.04763,0.528110872004958));
#9317=CARTESIAN_POINT('Ctrl Pts',(-0.528110872004958,-0.0476300000000001,
0.871530771444223));
#9318=CARTESIAN_POINT('Ctrl Pts',(-0.530395067942936,-0.0609922781173484,
0.87014664509073));
#9319=CARTESIAN_POINT('Ctrl Pts',(-0.533674141594226,-0.0742967091364493,
0.868149331745851));
#9320=CARTESIAN_POINT('Ctrl Pts',(-0.54708917182331,-0.115492077056649,
0.85981294420286));
#9321=CARTESIAN_POINT('Ctrl Pts',(-0.560922177770136,-0.141695629206859,
0.850993704737257));
#9322=CARTESIAN_POINT('Ctrl Pts',(-0.590422647829571,-0.181890537957859,
0.830754510485543));
#9323=CARTESIAN_POINT('Ctrl Pts',(-0.609616703125488,-0.201072148666545,
0.816896541396381));
#9324=CARTESIAN_POINT('Ctrl Pts',(-0.641117951819998,-0.223955109275652,
0.792310597819928));
#9325=CARTESIAN_POINT('Ctrl Pts',(-0.657208095763053,-0.232742381310829,
0.779109323683611));
#9326=CARTESIAN_POINT('Ctrl Pts',(-0.68964083160521,-0.244234834628584,
0.750552691816205));
#9327=CARTESIAN_POINT('Ctrl Pts',(-0.705971972091755,-0.246942143572133,
0.735185187071673));
#9328=CARTESIAN_POINT('Ctrl Pts',(-0.735185187071673,-0.246942143572133,
0.705971972091754));
#9329=CARTESIAN_POINT('Ctrl Pts',(-0.750552691816206,-0.244234834628584,
0.689640831605209));
#9330=CARTESIAN_POINT('Ctrl Pts',(-0.779109323683612,-0.232742381310829,
0.657208095763052));
#9331=CARTESIAN_POINT('Ctrl Pts',(-0.792310597819928,-0.223955109275652,
0.641117951819998));
#9332=CARTESIAN_POINT('Ctrl Pts',(-0.816896541396382,-0.201072148666545,
0.609616703125487));
#9333=CARTESIAN_POINT('Ctrl Pts',(-0.830754510485544,-0.181890537957858,
0.590422647829571));
#9334=CARTESIAN_POINT('Ctrl Pts',(-0.850993704737257,-0.141695629206858,
0.560922177770135));
#9335=CARTESIAN_POINT('Ctrl Pts',(-0.859812944202861,-0.115492077056649,
0.547089171823309));
#9336=CARTESIAN_POINT('Ctrl Pts',(-0.868149331745852,-0.0742967091364491,
0.533674141594226));
#9337=CARTESIAN_POINT('Ctrl Pts',(-0.870146645090731,-0.0609922781173483,
0.530395067942936));
#9338=CARTESIAN_POINT('Ctrl Pts',(-0.871530771444223,-0.04763,0.528110872004958));
#9339=CARTESIAN_POINT('',(-0.989696097314,-0.04763,0.242834539687906));
#9340=CARTESIAN_POINT('Origin',(0.,-0.04763,0.));
#9341=CARTESIAN_POINT('',(-1.019052,-0.246942143572133,1.248489836334E-16));
#9342=CARTESIAN_POINT('Ctrl Pts',(-0.989696097314,-0.04763,0.242834539687906));
#9343=CARTESIAN_POINT('Ctrl Pts',(-0.990332542620729,-0.0609922781173483,
0.24024064412003));
#9344=CARTESIAN_POINT('Ctrl Pts',(-0.991238884025248,-0.0742967091364492,
0.236509675094874));
#9345=CARTESIAN_POINT('Ctrl Pts',(-0.994830026707808,-0.115492077056649,
0.221129100087819));
#9346=CARTESIAN_POINT('Ctrl Pts',(-0.998375294985966,-0.141695629206859,
0.205111543747588));
#9347=CARTESIAN_POINT('Ctrl Pts',(-1.00492400591205,-0.181890537957859,
0.169940289819232));
#9348=CARTESIAN_POINT('Ctrl Pts',(-1.00869718865384,-0.201072148666545,
0.1465689792446));
#9349=CARTESIAN_POINT('Ctrl Pts',(-1.01358704779679,-0.223955109275652,
0.106909345252088));
#9350=CARTESIAN_POINT('Ctrl Pts',(-1.0156297872271,-0.232742381310829,0.0861971848975944));
#9351=CARTESIAN_POINT('Ctrl Pts',(-1.01837060663223,-0.244234834628584,
0.0430711894098825));
#9352=CARTESIAN_POINT('Ctrl Pts',(-1.019052,-0.246942143572133,0.0206568624125608));
#9353=CARTESIAN_POINT('Ctrl Pts',(-1.019052,-0.246942143572133,1.2490009027033E-16));
#9354=CARTESIAN_POINT('',(-1.019052,-0.28578,1.24797876996471E-16));
#9355=CARTESIAN_POINT('',(-1.019052,-0.166705,1.24797876996471E-16));
#9356=CARTESIAN_POINT('Origin',(0.,-0.28578,0.));
#9357=CARTESIAN_POINT('',(-0.989696097314,-0.04763,-0.242834539687906));
#9358=CARTESIAN_POINT('Ctrl Pts',(-1.019052,-0.246942143572133,1.2490009027033E-16));
#9359=CARTESIAN_POINT('Ctrl Pts',(-1.019052,-0.246942143572133,-0.0206568624125605));
#9360=CARTESIAN_POINT('Ctrl Pts',(-1.01837060663223,-0.244234834628584,
-0.0430711894098822));
#9361=CARTESIAN_POINT('Ctrl Pts',(-1.0156297872271,-0.232742381310829,-0.0861971848975941));
#9362=CARTESIAN_POINT('Ctrl Pts',(-1.01358704779679,-0.223955109275652,
-0.106909345252087));
#9363=CARTESIAN_POINT('Ctrl Pts',(-1.00869718865384,-0.201072148666546,
-0.1465689792446));
#9364=CARTESIAN_POINT('Ctrl Pts',(-1.00492400591205,-0.181890537957859,
-0.169940289819232));
#9365=CARTESIAN_POINT('Ctrl Pts',(-0.998375294985966,-0.141695629206859,
-0.205111543747588));
#9366=CARTESIAN_POINT('Ctrl Pts',(-0.994830026707808,-0.11549207705665,
-0.221129100087819));
#9367=CARTESIAN_POINT('Ctrl Pts',(-0.991238884025248,-0.0742967091364495,
-0.236509675094874));
#9368=CARTESIAN_POINT('Ctrl Pts',(-0.990332542620729,-0.0609922781173484,
-0.24024064412003));
#9369=CARTESIAN_POINT('Ctrl Pts',(-0.989696097314,-0.0476300000000001,-0.242834539687907));
#9370=CARTESIAN_POINT('',(-0.871530771444223,-0.04763,-0.528110872004958));
#9371=CARTESIAN_POINT('Origin',(0.,-0.04763,0.));
#9372=CARTESIAN_POINT('',(-0.528110872004958,-0.04763,-0.871530771444223));
#9373=CARTESIAN_POINT('Ctrl Pts',(-0.871530771444223,-0.0476300000000001,
-0.528110872004958));
#9374=CARTESIAN_POINT('Ctrl Pts',(-0.87014664509073,-0.0609922781173484,
-0.530395067942936));
#9375=CARTESIAN_POINT('Ctrl Pts',(-0.868149331745851,-0.0742967091364494,
-0.533674141594226));
#9376=CARTESIAN_POINT('Ctrl Pts',(-0.85981294420286,-0.115492077056649,
-0.54708917182331));
#9377=CARTESIAN_POINT('Ctrl Pts',(-0.850993704737257,-0.141695629206859,
-0.560922177770136));
#9378=CARTESIAN_POINT('Ctrl Pts',(-0.830754510485543,-0.181890537957859,
-0.590422647829571));
#9379=CARTESIAN_POINT('Ctrl Pts',(-0.816896541396381,-0.201072148666546,
-0.609616703125488));
#9380=CARTESIAN_POINT('Ctrl Pts',(-0.792310597819928,-0.223955109275652,
-0.641117951819999));
#9381=CARTESIAN_POINT('Ctrl Pts',(-0.779109323683611,-0.232742381310829,
-0.657208095763053));
#9382=CARTESIAN_POINT('Ctrl Pts',(-0.750552691816205,-0.244234834628584,
-0.68964083160521));
#9383=CARTESIAN_POINT('Ctrl Pts',(-0.735185187071673,-0.246942143572133,
-0.705971972091755));
#9384=CARTESIAN_POINT('Ctrl Pts',(-0.705971972091754,-0.246942143572133,
-0.735185187071673));
#9385=CARTESIAN_POINT('Ctrl Pts',(-0.68964083160521,-0.244234834628584,
-0.750552691816206));
#9386=CARTESIAN_POINT('Ctrl Pts',(-0.657208095763052,-0.232742381310829,
-0.779109323683612));
#9387=CARTESIAN_POINT('Ctrl Pts',(-0.641117951819998,-0.223955109275652,
-0.792310597819928));
#9388=CARTESIAN_POINT('Ctrl Pts',(-0.609616703125488,-0.201072148666545,
-0.816896541396381));
#9389=CARTESIAN_POINT('Ctrl Pts',(-0.590422647829571,-0.181890537957859,
-0.830754510485543));
#9390=CARTESIAN_POINT('Ctrl Pts',(-0.560922177770136,-0.141695629206859,
-0.850993704737257));
#9391=CARTESIAN_POINT('Ctrl Pts',(-0.54708917182331,-0.115492077056649,
-0.85981294420286));
#9392=CARTESIAN_POINT('Ctrl Pts',(-0.533674141594226,-0.0742967091364494,
-0.868149331745852));
#9393=CARTESIAN_POINT('Ctrl Pts',(-0.530395067942936,-0.0609922781173484,
-0.870146645090731));
#9394=CARTESIAN_POINT('Ctrl Pts',(-0.528110872004958,-0.0476300000000001,
-0.871530771444223));
#9395=CARTESIAN_POINT('',(-0.242834539687906,-0.04763,-0.989696097314));
#9396=CARTESIAN_POINT('Origin',(0.,-0.04763,0.));
#9397=CARTESIAN_POINT('',(0.242834539687906,-0.04763,-0.989696097314));
#9398=CARTESIAN_POINT('Ctrl Pts',(-0.242834539687907,-0.04763,-0.989696097314));
#9399=CARTESIAN_POINT('Ctrl Pts',(-0.24024064412003,-0.0609922781173483,
-0.990332542620729));
#9400=CARTESIAN_POINT('Ctrl Pts',(-0.236509675094874,-0.0742967091364493,
-0.991238884025248));
#9401=CARTESIAN_POINT('Ctrl Pts',(-0.221129100087819,-0.115492077056649,
-0.994830026707808));
#9402=CARTESIAN_POINT('Ctrl Pts',(-0.205111543747588,-0.141695629206859,
-0.998375294985966));
#9403=CARTESIAN_POINT('Ctrl Pts',(-0.169940289819232,-0.181890537957859,
-1.00492400591205));
#9404=CARTESIAN_POINT('Ctrl Pts',(-0.1465689792446,-0.201072148666545,-1.00869718865384));
#9405=CARTESIAN_POINT('Ctrl Pts',(-0.106909345252087,-0.223955109275652,
-1.01358704779679));
#9406=CARTESIAN_POINT('Ctrl Pts',(-0.0861971848975942,-0.232742381310829,
-1.0156297872271));
#9407=CARTESIAN_POINT('Ctrl Pts',(-0.0430711894098823,-0.244234834628584,
-1.01837060663223));
#9408=CARTESIAN_POINT('Ctrl Pts',(-0.0206568624125606,-0.246942143572133,
-1.019052));
#9409=CARTESIAN_POINT('Ctrl Pts',(0.0206568624125607,-0.246942143572133,
-1.019052));
#9410=CARTESIAN_POINT('Ctrl Pts',(0.0430711894098824,-0.244234834628584,
-1.01837060663223));
#9411=CARTESIAN_POINT('Ctrl Pts',(0.0861971848975943,-0.232742381310829,
-1.0156297872271));
#9412=CARTESIAN_POINT('Ctrl Pts',(0.106909345252088,-0.223955109275652,
-1.01358704779679));
#9413=CARTESIAN_POINT('Ctrl Pts',(0.1465689792446,-0.201072148666545,-1.00869718865384));
#9414=CARTESIAN_POINT('Ctrl Pts',(0.169940289819232,-0.181890537957859,
-1.00492400591205));
#9415=CARTESIAN_POINT('Ctrl Pts',(0.205111543747588,-0.141695629206859,
-0.998375294985966));
#9416=CARTESIAN_POINT('Ctrl Pts',(0.221129100087819,-0.115492077056649,
-0.994830026707808));
#9417=CARTESIAN_POINT('Ctrl Pts',(0.236509675094874,-0.0742967091364493,
-0.991238884025248));
#9418=CARTESIAN_POINT('Ctrl Pts',(0.24024064412003,-0.0609922781173484,
-0.990332542620729));
#9419=CARTESIAN_POINT('Ctrl Pts',(0.242834539687907,-0.04763,-0.989696097314));
#9420=CARTESIAN_POINT('',(0.528110872004958,-0.04763,-0.871530771444223));
#9421=CARTESIAN_POINT('Origin',(0.,-0.04763,0.));
#9422=CARTESIAN_POINT('',(0.871530771444223,-0.04763,-0.528110872004958));
#9423=CARTESIAN_POINT('Ctrl Pts',(0.528110872004958,-0.0476300000000001,
-0.871530771444223));
#9424=CARTESIAN_POINT('Ctrl Pts',(0.530395067942936,-0.0609922781173484,
-0.870146645090731));
#9425=CARTESIAN_POINT('Ctrl Pts',(0.533674141594226,-0.0742967091364493,
-0.868149331745851));
#9426=CARTESIAN_POINT('Ctrl Pts',(0.54708917182331,-0.115492077056649,-0.85981294420286));
#9427=CARTESIAN_POINT('Ctrl Pts',(0.560922177770136,-0.141695629206859,
-0.850993704737257));
#9428=CARTESIAN_POINT('Ctrl Pts',(0.590422647829571,-0.181890537957859,
-0.830754510485543));
#9429=CARTESIAN_POINT('Ctrl Pts',(0.609616703125488,-0.201072148666545,
-0.816896541396381));
#9430=CARTESIAN_POINT('Ctrl Pts',(0.641117951819998,-0.223955109275652,
-0.792310597819928));
#9431=CARTESIAN_POINT('Ctrl Pts',(0.657208095763053,-0.232742381310829,
-0.779109323683612));
#9432=CARTESIAN_POINT('Ctrl Pts',(0.68964083160521,-0.244234834628584,-0.750552691816206));
#9433=CARTESIAN_POINT('Ctrl Pts',(0.705971972091755,-0.246942143572133,
-0.735185187071673));
#9434=CARTESIAN_POINT('Ctrl Pts',(0.735185187071673,-0.246942143572133,
-0.705971972091754));
#9435=CARTESIAN_POINT('Ctrl Pts',(0.750552691816206,-0.244234834628584,
-0.68964083160521));
#9436=CARTESIAN_POINT('Ctrl Pts',(0.779109323683612,-0.232742381310829,
-0.657208095763053));
#9437=CARTESIAN_POINT('Ctrl Pts',(0.792310597819928,-0.223955109275652,
-0.641117951819998));
#9438=CARTESIAN_POINT('Ctrl Pts',(0.816896541396381,-0.201072148666545,
-0.609616703125488));
#9439=CARTESIAN_POINT('Ctrl Pts',(0.830754510485543,-0.181890537957859,
-0.590422647829571));
#9440=CARTESIAN_POINT('Ctrl Pts',(0.850993704737257,-0.141695629206859,
-0.560922177770136));
#9441=CARTESIAN_POINT('Ctrl Pts',(0.85981294420286,-0.115492077056649,-0.54708917182331));
#9442=CARTESIAN_POINT('Ctrl Pts',(0.868149331745851,-0.0742967091364493,
-0.533674141594226));
#9443=CARTESIAN_POINT('Ctrl Pts',(0.870146645090731,-0.0609922781173484,
-0.530395067942936));
#9444=CARTESIAN_POINT('Ctrl Pts',(0.871530771444223,-0.0476300000000001,
-0.528110872004958));
#9445=CARTESIAN_POINT('',(0.989696097314,-0.04763,-0.242834539687906));
#9446=CARTESIAN_POINT('Origin',(0.,-0.04763,0.));
#9447=CARTESIAN_POINT('',(0.989696097314,-0.04763,0.242834539687906));
#9448=CARTESIAN_POINT('Ctrl Pts',(0.989696097314,-0.04763,-0.242834539687907));
#9449=CARTESIAN_POINT('Ctrl Pts',(0.990332542620729,-0.0609922781173483,
-0.24024064412003));
#9450=CARTESIAN_POINT('Ctrl Pts',(0.991238884025248,-0.0742967091364493,
-0.236509675094874));
#9451=CARTESIAN_POINT('Ctrl Pts',(0.994830026707808,-0.115492077056649,
-0.221129100087819));
#9452=CARTESIAN_POINT('Ctrl Pts',(0.998375294985966,-0.141695629206859,
-0.205111543747588));
#9453=CARTESIAN_POINT('Ctrl Pts',(1.00492400591205,-0.181890537957859,-0.169940289819232));
#9454=CARTESIAN_POINT('Ctrl Pts',(1.00869718865384,-0.201072148666545,-0.1465689792446));
#9455=CARTESIAN_POINT('Ctrl Pts',(1.01358704779679,-0.223955109275652,-0.106909345252087));
#9456=CARTESIAN_POINT('Ctrl Pts',(1.0156297872271,-0.232742381310829,-0.0861971848975942));
#9457=CARTESIAN_POINT('Ctrl Pts',(1.01837060663223,-0.244234834628584,-0.0430711894098823));
#9458=CARTESIAN_POINT('Ctrl Pts',(1.019052,-0.246942143572133,-0.0206568624125607));
#9459=CARTESIAN_POINT('Ctrl Pts',(1.019052,-0.246942143572133,0.0206568624125607));
#9460=CARTESIAN_POINT('Ctrl Pts',(1.01837060663223,-0.244234834628584,0.0430711894098823));
#9461=CARTESIAN_POINT('Ctrl Pts',(1.0156297872271,-0.232742381310829,0.0861971848975942));
#9462=CARTESIAN_POINT('Ctrl Pts',(1.01358704779679,-0.223955109275652,0.106909345252087));
#9463=CARTESIAN_POINT('Ctrl Pts',(1.00869718865384,-0.201072148666545,0.1465689792446));
#9464=CARTESIAN_POINT('Ctrl Pts',(1.00492400591205,-0.181890537957859,0.169940289819232));
#9465=CARTESIAN_POINT('Ctrl Pts',(0.998375294985966,-0.141695629206859,
0.205111543747588));
#9466=CARTESIAN_POINT('Ctrl Pts',(0.994830026707808,-0.115492077056649,
0.221129100087819));
#9467=CARTESIAN_POINT('Ctrl Pts',(0.991238884025248,-0.0742967091364492,
0.236509675094874));
#9468=CARTESIAN_POINT('Ctrl Pts',(0.990332542620729,-0.0609922781173483,
0.24024064412003));
#9469=CARTESIAN_POINT('Ctrl Pts',(0.989696097314,-0.04763,0.242834539687907));
#9470=CARTESIAN_POINT('Origin',(0.,-0.04763,0.));
#9471=CARTESIAN_POINT('Origin',(0.,-0.04763,0.));
#9472=CARTESIAN_POINT('',(0.238183666596899,-0.04763,0.951592097314));
#9473=CARTESIAN_POINT('Origin',(0.,-0.04763,0.));
#9474=CARTESIAN_POINT('Origin',(-1.94289029309402E-16,-0.04763,1.));
#9475=CARTESIAN_POINT('Origin',(-1.94289029309402E-16,0.,1.));
#9476=CARTESIAN_POINT('',(-0.2381836665969,-0.04763,0.951592097314));
#9477=CARTESIAN_POINT('Ctrl Pts',(-0.238183666596899,-0.0476299999999999,
0.951592097314));
#9478=CARTESIAN_POINT('Ctrl Pts',(-0.233157223576062,-0.0740444353928835,
0.952850216871763));
#9479=CARTESIAN_POINT('Ctrl Pts',(-0.223801617934946,-0.0999305678883309,
0.955173119738174));
#9480=CARTESIAN_POINT('Ctrl Pts',(-0.199966927975188,-0.142345102874864,
0.960411259488514));
#9481=CARTESIAN_POINT('Ctrl Pts',(-0.1868781821531,-0.159766064500479,0.963103647174702));
#9482=CARTESIAN_POINT('Ctrl Pts',(-0.15681442133453,-0.190326085855194,
0.968453058988463));
#9483=CARTESIAN_POINT('Ctrl Pts',(-0.139836317888043,-0.203463743702801,
0.971100730005489));
#9484=CARTESIAN_POINT('Ctrl Pts',(-0.104422493053067,-0.224161999508995,
0.975530745318961));
#9485=CARTESIAN_POINT('Ctrl Pts',(-0.0842175114474176,-0.232861760990032,
0.977553872336861));
#9486=CARTESIAN_POINT('Ctrl Pts',(-0.0421062857595701,-0.244251601209411,
0.980270995488453));
#9487=CARTESIAN_POINT('Ctrl Pts',(-0.0201990724523197,-0.246942143572133,
0.980948));
#9488=CARTESIAN_POINT('Ctrl Pts',(0.020199072452319,-0.246942143572133,
0.980948));
#9489=CARTESIAN_POINT('Ctrl Pts',(0.0421062857595694,-0.244251601209411,
0.980270995488454));
#9490=CARTESIAN_POINT('Ctrl Pts',(0.0842175114474169,-0.232861760990032,
0.977553872336861));
#9491=CARTESIAN_POINT('Ctrl Pts',(0.104422493053067,-0.224161999508995,
0.975530745318961));
#9492=CARTESIAN_POINT('Ctrl Pts',(0.139836317888042,-0.203463743702801,
0.971100730005489));
#9493=CARTESIAN_POINT('Ctrl Pts',(0.15681442133453,-0.190326085855194,0.968453058988463));
#9494=CARTESIAN_POINT('Ctrl Pts',(0.1868781821531,-0.15976606450048,0.963103647174702));
#9495=CARTESIAN_POINT('Ctrl Pts',(0.199966927975188,-0.142345102874864,
0.960411259488514));
#9496=CARTESIAN_POINT('Ctrl Pts',(0.223801617934945,-0.0999305678883309,
0.955173119738174));
#9497=CARTESIAN_POINT('Ctrl Pts',(0.233157223576061,-0.0740444353928835,
0.952850216871763));
#9498=CARTESIAN_POINT('Ctrl Pts',(0.238183666596899,-0.0476299999999999,
0.951592097314));
#9499=CARTESIAN_POINT('Origin',(-1.94289029309402E-16,-0.04763,1.));
#9500=CARTESIAN_POINT('Origin',(0.,-0.04763,0.));
#9501=CARTESIAN_POINT('',(-0.504455939115715,-0.04763,0.841298510752802));
#9502=CARTESIAN_POINT('Origin',(0.,-0.04763,0.));
#9503=CARTESIAN_POINT('Origin',(-0.707106781186548,-0.04763,0.707106781186547));
#9504=CARTESIAN_POINT('Origin',(-0.707106781186548,0.,0.707106781186547));
#9505=CARTESIAN_POINT('',(-0.841298510752802,-0.04763,0.504455939115715));
#9506=CARTESIAN_POINT('Ctrl Pts',(-0.841298510752802,-0.04763,0.504455939115715));
#9507=CARTESIAN_POINT('Ctrl Pts',(-0.838633903678357,-0.0740444353928835,
0.508899795931835));
#9508=CARTESIAN_POINT('Ctrl Pts',(-0.833661031856294,-0.0999305678883309,
0.517157748491652));
#9509=CARTESIAN_POINT('Ctrl Pts',(-0.820511285096538,-0.142345102874864,
0.537715343527944));
#9510=CARTESIAN_POINT('Ctrl Pts',(-0.813159949759,-0.159766064500479,0.548874290046456));
#9511=CARTESIAN_POINT('Ctrl Pts',(-0.795684265985089,-0.190326085855194,
0.573915184558107));
#9512=CARTESIAN_POINT('Ctrl Pts',(-0.78555112003688,-0.203463743702801,
0.587792702767295));
#9513=CARTESIAN_POINT('Ctrl Pts',(-0.763642258217233,-0.224161999508995,
0.615966552324775));
#9514=CARTESIAN_POINT('Ctrl Pts',(-0.750785745543687,-0.232861760990032,
0.631684198665438));
#9515=CARTESIAN_POINT('Ctrl Pts',(-0.722929908501543,-0.244251601209411,
0.663382628119203));
#9516=CARTESIAN_POINT('Ctrl Pts',(-0.707917883896095,-0.246942143572133,
0.679352081686668));
#9517=CARTESIAN_POINT('Ctrl Pts',(-0.679352081686668,-0.246942143572133,
0.707917883896095));
#9518=CARTESIAN_POINT('Ctrl Pts',(-0.663382628119203,-0.244251601209411,
0.722929908501544));
#9519=CARTESIAN_POINT('Ctrl Pts',(-0.631684198665438,-0.232861760990031,
0.750785745543687));
#9520=CARTESIAN_POINT('Ctrl Pts',(-0.615966552324775,-0.224161999508995,
0.763642258217233));
#9521=CARTESIAN_POINT('Ctrl Pts',(-0.587792702767295,-0.203463743702801,
0.78555112003688));
#9522=CARTESIAN_POINT('Ctrl Pts',(-0.573915184558107,-0.190326085855194,
0.795684265985088));
#9523=CARTESIAN_POINT('Ctrl Pts',(-0.548874290046456,-0.159766064500479,
0.813159949759));
#9524=CARTESIAN_POINT('Ctrl Pts',(-0.537715343527944,-0.142345102874864,
0.820511285096538));
#9525=CARTESIAN_POINT('Ctrl Pts',(-0.517157748491652,-0.0999305678883309,
0.833661031856294));
#9526=CARTESIAN_POINT('Ctrl Pts',(-0.508899795931835,-0.0740444353928835,
0.838633903678357));
#9527=CARTESIAN_POINT('Ctrl Pts',(-0.504455939115716,-0.04763,0.841298510752801));
#9528=CARTESIAN_POINT('Origin',(-0.707106781186548,-0.04763,0.707106781186547));
#9529=CARTESIAN_POINT('Origin',(0.,-0.04763,0.));
#9530=CARTESIAN_POINT('',(-0.951592097314,-0.04763,0.238183666596899));
#9531=CARTESIAN_POINT('Origin',(0.,-0.04763,0.));
#9532=CARTESIAN_POINT('Origin',(-1.,-0.04763,-1.11022302462516E-16));
#9533=CARTESIAN_POINT('Origin',(-1.,0.,-1.11022302462516E-16));
#9534=CARTESIAN_POINT('',(-0.951592097314,-0.04763,-0.2381836665969));
#9535=CARTESIAN_POINT('',(-0.980948,-0.246942143572133,1.08514323328844E-18));
#9536=CARTESIAN_POINT('Ctrl Pts',(-0.951592097314,-0.04763,-0.238183666596899));
#9537=CARTESIAN_POINT('Ctrl Pts',(-0.952850216871763,-0.0740444353928835,
-0.233157223576062));
#9538=CARTESIAN_POINT('Ctrl Pts',(-0.955173119738174,-0.0999305678883309,
-0.223801617934946));
#9539=CARTESIAN_POINT('Ctrl Pts',(-0.960411259488514,-0.142345102874864,
-0.199966927975188));
#9540=CARTESIAN_POINT('Ctrl Pts',(-0.963103647174702,-0.159766064500479,
-0.1868781821531));
#9541=CARTESIAN_POINT('Ctrl Pts',(-0.968453058988463,-0.190326085855194,
-0.15681442133453));
#9542=CARTESIAN_POINT('Ctrl Pts',(-0.971100730005489,-0.203463743702801,
-0.139836317888043));
#9543=CARTESIAN_POINT('Ctrl Pts',(-0.975530745318961,-0.224161999508995,
-0.104422493053067));
#9544=CARTESIAN_POINT('Ctrl Pts',(-0.977553872336861,-0.232861760990032,
-0.0842175114474175));
#9545=CARTESIAN_POINT('Ctrl Pts',(-0.980270995488453,-0.244251601209411,
-0.0421062857595699));
#9546=CARTESIAN_POINT('Ctrl Pts',(-0.980948,-0.246942143572133,-0.0201990724523195));
#9547=CARTESIAN_POINT('Ctrl Pts',(-0.980948,-0.246942143572133,-1.17961196366423E-16));
#9548=CARTESIAN_POINT('Origin',(-1.,-0.04763,-1.11022302462516E-16));
#9549=CARTESIAN_POINT('Ctrl Pts',(-0.980948,-0.246942143572133,-1.17961196366423E-16));
#9550=CARTESIAN_POINT('Ctrl Pts',(-0.980948,-0.246942143572133,0.0201990724523192));
#9551=CARTESIAN_POINT('Ctrl Pts',(-0.980270995488453,-0.244251601209411,
0.0421062857595695));
#9552=CARTESIAN_POINT('Ctrl Pts',(-0.977553872336861,-0.232861760990032,
0.0842175114474169));
#9553=CARTESIAN_POINT('Ctrl Pts',(-0.975530745318961,-0.224161999508995,
0.104422493053066));
#9554=CARTESIAN_POINT('Ctrl Pts',(-0.971100730005489,-0.203463743702801,
0.139836317888042));
#9555=CARTESIAN_POINT('Ctrl Pts',(-0.968453058988463,-0.190326085855194,
0.15681442133453));
#9556=CARTESIAN_POINT('Ctrl Pts',(-0.963103647174702,-0.15976606450048,
0.1868781821531));
#9557=CARTESIAN_POINT('Ctrl Pts',(-0.960411259488514,-0.142345102874864,
0.199966927975188));
#9558=CARTESIAN_POINT('Ctrl Pts',(-0.955173119738174,-0.099930567888331,
0.223801617934945));
#9559=CARTESIAN_POINT('Ctrl Pts',(-0.952850216871763,-0.0740444353928835,
0.233157223576061));
#9560=CARTESIAN_POINT('Ctrl Pts',(-0.951592097314,-0.04763,0.238183666596899));
#9561=CARTESIAN_POINT('Origin',(0.,-0.04763,0.));
#9562=CARTESIAN_POINT('',(-0.841298510752802,-0.04763,-0.504455939115715));
#9563=CARTESIAN_POINT('Origin',(0.,-0.04763,0.));
#9564=CARTESIAN_POINT('Origin',(-0.707106781186547,-0.04763,-0.707106781186548));
#9565=CARTESIAN_POINT('Origin',(-0.707106781186547,0.,-0.707106781186548));
#9566=CARTESIAN_POINT('',(-0.504455939115715,-0.04763,-0.841298510752802));
#9567=CARTESIAN_POINT('Ctrl Pts',(-0.504455939115715,-0.04763,-0.841298510752802));
#9568=CARTESIAN_POINT('Ctrl Pts',(-0.508899795931835,-0.0740444353928835,
-0.838633903678357));
#9569=CARTESIAN_POINT('Ctrl Pts',(-0.517157748491652,-0.0999305678883309,
-0.833661031856294));
#9570=CARTESIAN_POINT('Ctrl Pts',(-0.537715343527944,-0.142345102874864,
-0.820511285096538));
#9571=CARTESIAN_POINT('Ctrl Pts',(-0.548874290046456,-0.159766064500479,
-0.813159949759));
#9572=CARTESIAN_POINT('Ctrl Pts',(-0.573915184558107,-0.190326085855194,
-0.795684265985089));
#9573=CARTESIAN_POINT('Ctrl Pts',(-0.587792702767295,-0.203463743702801,
-0.78555112003688));
#9574=CARTESIAN_POINT('Ctrl Pts',(-0.615966552324775,-0.224161999508995,
-0.763642258217233));
#9575=CARTESIAN_POINT('Ctrl Pts',(-0.631684198665438,-0.232861760990032,
-0.750785745543687));
#9576=CARTESIAN_POINT('Ctrl Pts',(-0.663382628119203,-0.244251601209411,
-0.722929908501543));
#9577=CARTESIAN_POINT('Ctrl Pts',(-0.679352081686668,-0.246942143572133,
-0.707917883896095));
#9578=CARTESIAN_POINT('Ctrl Pts',(-0.707917883896095,-0.246942143572133,
-0.679352081686668));
#9579=CARTESIAN_POINT('Ctrl Pts',(-0.722929908501543,-0.244251601209411,
-0.663382628119203));
#9580=CARTESIAN_POINT('Ctrl Pts',(-0.750785745543687,-0.232861760990032,
-0.631684198665439));
#9581=CARTESIAN_POINT('Ctrl Pts',(-0.763642258217232,-0.224161999508995,
-0.615966552324775));
#9582=CARTESIAN_POINT('Ctrl Pts',(-0.78555112003688,-0.203463743702801,
-0.587792702767295));
#9583=CARTESIAN_POINT('Ctrl Pts',(-0.795684265985088,-0.190326085855194,
-0.573915184558107));
#9584=CARTESIAN_POINT('Ctrl Pts',(-0.813159949759,-0.15976606450048,-0.548874290046456));
#9585=CARTESIAN_POINT('Ctrl Pts',(-0.820511285096538,-0.142345102874864,
-0.537715343527944));
#9586=CARTESIAN_POINT('Ctrl Pts',(-0.833661031856294,-0.0999305678883311,
-0.517157748491652));
#9587=CARTESIAN_POINT('Ctrl Pts',(-0.838633903678357,-0.0740444353928836,
-0.508899795931835));
#9588=CARTESIAN_POINT('Ctrl Pts',(-0.841298510752801,-0.04763,-0.504455939115715));
#9589=CARTESIAN_POINT('Origin',(-0.707106781186547,-0.04763,-0.707106781186548));
#9590=CARTESIAN_POINT('Origin',(0.,-0.04763,0.));
#9591=CARTESIAN_POINT('',(-0.238183666596899,-0.04763,-0.951592097314));
#9592=CARTESIAN_POINT('Origin',(0.,-0.04763,0.));
#9593=CARTESIAN_POINT('Origin',(5.55111512312578E-17,-0.04763,-1.));
#9594=CARTESIAN_POINT('Origin',(5.55111512312578E-17,0.,-1.));
#9595=CARTESIAN_POINT('',(0.238183666596899,-0.04763,-0.951592097314));
#9596=CARTESIAN_POINT('Ctrl Pts',(0.238183666596899,-0.04763,-0.951592097314));
#9597=CARTESIAN_POINT('Ctrl Pts',(0.233157223576062,-0.0740444353928835,
-0.952850216871763));
#9598=CARTESIAN_POINT('Ctrl Pts',(0.223801617934946,-0.099930567888331,
-0.955173119738174));
#9599=CARTESIAN_POINT('Ctrl Pts',(0.199966927975188,-0.142345102874864,
-0.960411259488514));
#9600=CARTESIAN_POINT('Ctrl Pts',(0.1868781821531,-0.15976606450048,-0.963103647174702));
#9601=CARTESIAN_POINT('Ctrl Pts',(0.15681442133453,-0.190326085855194,-0.968453058988463));
#9602=CARTESIAN_POINT('Ctrl Pts',(0.139836317888042,-0.203463743702801,
-0.971100730005489));
#9603=CARTESIAN_POINT('Ctrl Pts',(0.104422493053067,-0.224161999508995,
-0.975530745318961));
#9604=CARTESIAN_POINT('Ctrl Pts',(0.0842175114474173,-0.232861760990032,
-0.977553872336861));
#9605=CARTESIAN_POINT('Ctrl Pts',(0.0421062857595698,-0.244251601209411,
-0.980270995488453));
#9606=CARTESIAN_POINT('Ctrl Pts',(0.0201990724523194,-0.246942143572133,
-0.980948));
#9607=CARTESIAN_POINT('Ctrl Pts',(-0.0201990724523193,-0.246942143572133,
-0.980948));
#9608=CARTESIAN_POINT('Ctrl Pts',(-0.0421062857595697,-0.244251601209411,
-0.980270995488453));
#9609=CARTESIAN_POINT('Ctrl Pts',(-0.0842175114474171,-0.232861760990032,
-0.977553872336861));
#9610=CARTESIAN_POINT('Ctrl Pts',(-0.104422493053067,-0.224161999508995,
-0.975530745318961));
#9611=CARTESIAN_POINT('Ctrl Pts',(-0.139836317888042,-0.203463743702801,
-0.971100730005489));
#9612=CARTESIAN_POINT('Ctrl Pts',(-0.15681442133453,-0.190326085855194,
-0.968453058988463));
#9613=CARTESIAN_POINT('Ctrl Pts',(-0.1868781821531,-0.15976606450048,-0.963103647174702));
#9614=CARTESIAN_POINT('Ctrl Pts',(-0.199966927975188,-0.142345102874864,
-0.960411259488514));
#9615=CARTESIAN_POINT('Ctrl Pts',(-0.223801617934945,-0.099930567888331,
-0.955173119738174));
#9616=CARTESIAN_POINT('Ctrl Pts',(-0.233157223576062,-0.0740444353928835,
-0.952850216871763));
#9617=CARTESIAN_POINT('Ctrl Pts',(-0.238183666596899,-0.0476299999999999,
-0.951592097314));
#9618=CARTESIAN_POINT('Origin',(5.55111512312578E-17,-0.04763,-1.));
#9619=CARTESIAN_POINT('Origin',(0.,-0.04763,0.));
#9620=CARTESIAN_POINT('',(0.504455939115715,-0.04763,-0.841298510752802));
#9621=CARTESIAN_POINT('Origin',(0.,-0.04763,0.));
#9622=CARTESIAN_POINT('Origin',(0.707106781186548,-0.04763,-0.707106781186547));
#9623=CARTESIAN_POINT('Origin',(0.707106781186548,0.,-0.707106781186547));
#9624=CARTESIAN_POINT('',(0.841298510752802,-0.04763,-0.504455939115715));
#9625=CARTESIAN_POINT('Ctrl Pts',(0.841298510752802,-0.04763,-0.504455939115715));
#9626=CARTESIAN_POINT('Ctrl Pts',(0.838633903678357,-0.0740444353928835,
-0.508899795931835));
#9627=CARTESIAN_POINT('Ctrl Pts',(0.833661031856294,-0.0999305678883309,
-0.517157748491652));
#9628=CARTESIAN_POINT('Ctrl Pts',(0.820511285096538,-0.142345102874864,
-0.537715343527944));
#9629=CARTESIAN_POINT('Ctrl Pts',(0.813159949759,-0.159766064500479,-0.548874290046456));
#9630=CARTESIAN_POINT('Ctrl Pts',(0.795684265985088,-0.190326085855194,
-0.573915184558107));
#9631=CARTESIAN_POINT('Ctrl Pts',(0.78555112003688,-0.203463743702801,-0.587792702767295));
#9632=CARTESIAN_POINT('Ctrl Pts',(0.763642258217233,-0.224161999508995,
-0.615966552324775));
#9633=CARTESIAN_POINT('Ctrl Pts',(0.750785745543687,-0.232861760990032,
-0.631684198665438));
#9634=CARTESIAN_POINT('Ctrl Pts',(0.722929908501543,-0.244251601209411,
-0.663382628119203));
#9635=CARTESIAN_POINT('Ctrl Pts',(0.707917883896095,-0.246942143572133,
-0.679352081686668));
#9636=CARTESIAN_POINT('Ctrl Pts',(0.679352081686668,-0.246942143572133,
-0.707917883896095));
#9637=CARTESIAN_POINT('Ctrl Pts',(0.663382628119203,-0.244251601209411,
-0.722929908501543));
#9638=CARTESIAN_POINT('Ctrl Pts',(0.631684198665438,-0.232861760990032,
-0.750785745543687));
#9639=CARTESIAN_POINT('Ctrl Pts',(0.615966552324775,-0.224161999508995,
-0.763642258217232));
#9640=CARTESIAN_POINT('Ctrl Pts',(0.587792702767295,-0.203463743702801,
-0.78555112003688));
#9641=CARTESIAN_POINT('Ctrl Pts',(0.573915184558107,-0.190326085855194,
-0.795684265985088));
#9642=CARTESIAN_POINT('Ctrl Pts',(0.548874290046456,-0.159766064500479,
-0.813159949759));
#9643=CARTESIAN_POINT('Ctrl Pts',(0.537715343527944,-0.142345102874864,
-0.820511285096538));
#9644=CARTESIAN_POINT('Ctrl Pts',(0.517157748491652,-0.099930567888331,
-0.833661031856294));
#9645=CARTESIAN_POINT('Ctrl Pts',(0.508899795931835,-0.0740444353928835,
-0.838633903678357));
#9646=CARTESIAN_POINT('Ctrl Pts',(0.504455939115715,-0.04763,-0.841298510752801));
#9647=CARTESIAN_POINT('Origin',(0.707106781186548,-0.04763,-0.707106781186547));
#9648=CARTESIAN_POINT('Origin',(0.,-0.166705,0.));
#9649=CARTESIAN_POINT('',(-0.980948,-0.28578,1.20131482833E-16));
#9650=CARTESIAN_POINT('Origin',(0.,-0.28578,0.));
#9651=CARTESIAN_POINT('',(-0.980948,-0.166705,1.20131482833E-16));
#9652=CARTESIAN_POINT('',(0.951592097314,-0.04763,0.238183666596899));
#9653=CARTESIAN_POINT('Origin',(0.,-0.04763,0.));
#9654=CARTESIAN_POINT('',(0.951592097314,-0.04763,-0.238183666596899));
#9655=CARTESIAN_POINT('Ctrl Pts',(0.951592097314,-0.04763,0.238183666596899));
#9656=CARTESIAN_POINT('Ctrl Pts',(0.952850216871763,-0.0740444353928835,
0.233157223576062));
#9657=CARTESIAN_POINT('Ctrl Pts',(0.955173119738174,-0.099930567888331,
0.223801617934945));
#9658=CARTESIAN_POINT('Ctrl Pts',(0.960411259488514,-0.142345102874864,
0.199966927975188));
#9659=CARTESIAN_POINT('Ctrl Pts',(0.963103647174702,-0.15976606450048,0.1868781821531));
#9660=CARTESIAN_POINT('Ctrl Pts',(0.968453058988463,-0.190326085855194,
0.15681442133453));
#9661=CARTESIAN_POINT('Ctrl Pts',(0.971100730005489,-0.203463743702801,
0.139836317888042));
#9662=CARTESIAN_POINT('Ctrl Pts',(0.975530745318961,-0.224161999508995,
0.104422493053067));
#9663=CARTESIAN_POINT('Ctrl Pts',(0.977553872336861,-0.232861760990032,
0.0842175114474172));
#9664=CARTESIAN_POINT('Ctrl Pts',(0.980270995488453,-0.244251601209411,
0.0421062857595697));
#9665=CARTESIAN_POINT('Ctrl Pts',(0.980948,-0.246942143572133,0.0201990724523194));
#9666=CARTESIAN_POINT('Ctrl Pts',(0.980948,-0.246942143572133,-0.0201990724523194));
#9667=CARTESIAN_POINT('Ctrl Pts',(0.980270995488453,-0.244251601209411,
-0.0421062857595697));
#9668=CARTESIAN_POINT('Ctrl Pts',(0.977553872336861,-0.232861760990032,
-0.0842175114474172));
#9669=CARTESIAN_POINT('Ctrl Pts',(0.975530745318961,-0.224161999508995,
-0.104422493053067));
#9670=CARTESIAN_POINT('Ctrl Pts',(0.971100730005489,-0.203463743702801,
-0.139836317888042));
#9671=CARTESIAN_POINT('Ctrl Pts',(0.968453058988463,-0.190326085855194,
-0.15681442133453));
#9672=CARTESIAN_POINT('Ctrl Pts',(0.963103647174702,-0.15976606450048,-0.1868781821531));
#9673=CARTESIAN_POINT('Ctrl Pts',(0.960411259488514,-0.142345102874864,
-0.199966927975188));
#9674=CARTESIAN_POINT('Ctrl Pts',(0.955173119738174,-0.099930567888331,
-0.223801617934945));
#9675=CARTESIAN_POINT('Ctrl Pts',(0.952850216871763,-0.0740444353928835,
-0.233157223576062));
#9676=CARTESIAN_POINT('Ctrl Pts',(0.951592097314,-0.0476299999999999,-0.238183666596899));
#9677=CARTESIAN_POINT('Origin',(0.,-0.04763,0.));
#9678=CARTESIAN_POINT('Origin',(0.,-0.04763,0.));
#9679=CARTESIAN_POINT('Origin',(1.,-0.04763,0.));
#9680=CARTESIAN_POINT('Origin',(1.,0.,0.));
#9681=CARTESIAN_POINT('Origin',(1.,-0.04763,0.));
#9682=CARTESIAN_POINT('Origin',(0.,-0.28578,0.));
#9683=CARTESIAN_POINT('Origin',(0.,-0.04763,0.));
#10790=UNCERTAINTY_MEASURE_WITH_UNIT(LENGTH_MEASURE(0.001),#10838,
'DISTANCE_ACCURACY_VALUE',
'Maximum model space distance between geometric entities at asserted c
onnectivities');
#10807=UNCERTAINTY_MEASURE_WITH_UNIT(LENGTH_MEASURE(0.001),#10838,
'DISTANCE_ACCURACY_VALUE',
'Maximum model space distance between geometric entities at asserted c
onnectivities');
#10820=(
GEOMETRIC_REPRESENTATION_CONTEXT(3)
GLOBAL_UNCERTAINTY_ASSIGNED_CONTEXT((#10790))
GLOBAL_UNIT_ASSIGNED_CONTEXT((#10838,#10840,#10841))
REPRESENTATION_CONTEXT('','3D')
);
#10837=(
GEOMETRIC_REPRESENTATION_CONTEXT(3)
GLOBAL_UNCERTAINTY_ASSIGNED_CONTEXT((#10807))
GLOBAL_UNIT_ASSIGNED_CONTEXT((#10838,#10840,#10841))
REPRESENTATION_CONTEXT('','3D')
);
#10838=(
LENGTH_UNIT()
NAMED_UNIT(*)
SI_UNIT(.CENTI.,.METRE.)
);
#10840=(
NAMED_UNIT(*)
PLANE_ANGLE_UNIT()
SI_UNIT($,.RADIAN.)
);
#10841=(
NAMED_UNIT(*)
SI_UNIT($,.STERADIAN.)
SOLID_ANGLE_UNIT()
);
#10854=SHAPE_DEFINITION_REPRESENTATION(#10883,#10953);
#10883=PRODUCT_DEFINITION_SHAPE('',$,#10983);
#10953=SHAPE_REPRESENTATION('',(#6246),#10820);
#10970=PRODUCT_DEFINITION_CONTEXT('part definition',#11059,'design');
#10983=PRODUCT_DEFINITION('Cage','Cage',#11012,#10970);
#11012=PRODUCT_DEFINITION_FORMATION('',$,#11073);
#11059=APPLICATION_CONTEXT(
'Core Data for Automotive Mechanical Design Process');
#11060=PRODUCT_CONTEXT('part definition',#11059,'mechanical');
#11073=PRODUCT('Cage','Cage','Cage',(#11060));
#11160=COLOUR_RGB('Grey',0.48,0.52,0.57);
#11161=FILL_AREA_STYLE_COLOUR('',#11160);
#11162=FILL_AREA_STYLE('',(#11161));
#11163=SURFACE_STYLE_FILL_AREA(#11162);
#11164=SURFACE_SIDE_STYLE('',(#11163));
#11165=SURFACE_STYLE_USAGE(.BOTH.,#11164);
#11166=PRESENTATION_STYLE_ASSIGNMENT((#11165));
ENDSEC;
END-ISO-10303-21;
